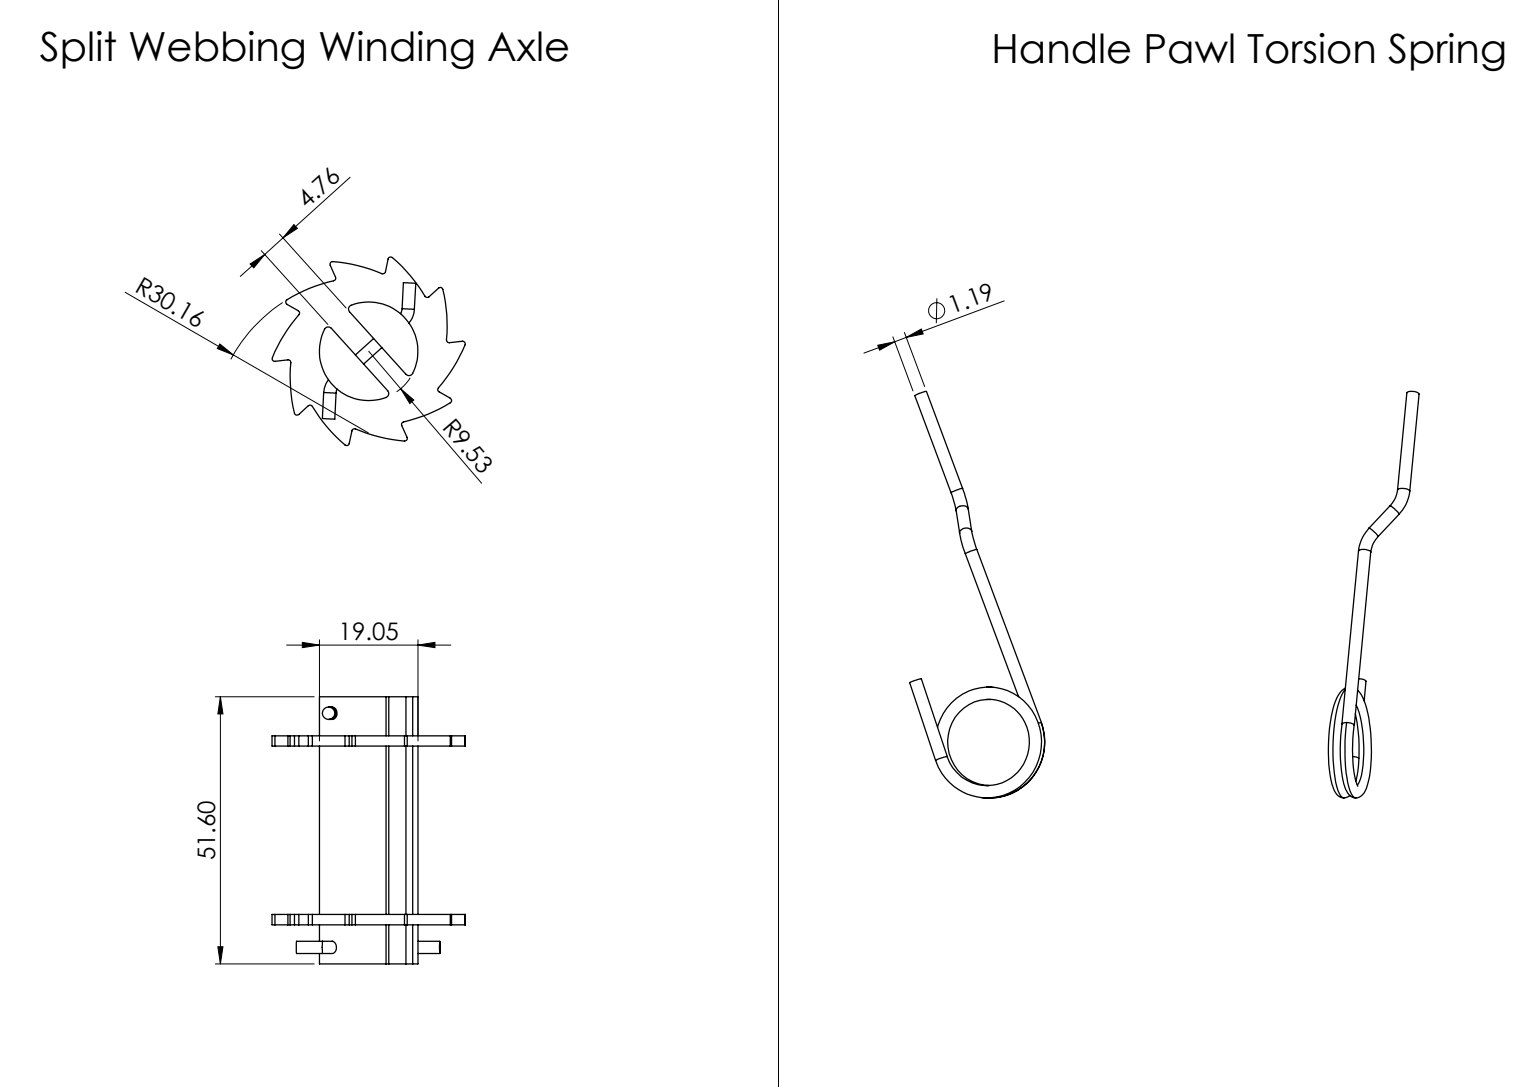
ISO-10303-21;
HEADER;
FILE_DESCRIPTION (('STEP AP214'),
    '1' );
FILE_NAME ('Handle Pawl Torsion Spring.step',
    '2026-10-09T14:10:49',
    ( '' ),
    ( '' ),
    'SwSTEP 2.0',
    'SolidWorks 2026',
    '' );
FILE_SCHEMA (( 'AUTOMOTIVE_DESIGN' ));
ENDSEC;

DATA;
#16=CARTESIAN_POINT ( 'NONE',  ( 20.19277141636333894, -1.028702071915735816, -14.77014087419847499 ) ) ;
#19=CARTESIAN_POINT ( 'NONE',  ( 10.74587282237300023, -3.551474423027108696, -17.13904648846254730 ) ) ;
#30=CARTESIAN_POINT ( 'NONE',  ( 16.87573345534896063, 1.342421174834532049, -14.70424319714138583 ) ) ;
#38=ADVANCED_FACE ( 'NONE', ( #13541 ), #20247, .T. ) ;
#40=CLOSED_SHELL ( 'NONE', ( #13341, #4807, #5036, #2626, #8435, #8593, #10298, #38, #14436, #19908, #617, #19403, #13246, #15792, #17350, #9101 ) ) ;
#47=CARTESIAN_POINT ( 'NONE',  ( 12.03790632155779505, -1.842118199788904453, -16.73074338374886594 ) ) ;
#86=CARTESIAN_POINT ( 'NONE',  ( 19.20082524333561125, -5.215953177437151034, -14.22689379871408022 ) ) ;
#131=CARTESIAN_POINT ( 'NONE',  ( 19.71883509336728224, 0.07040483093252521141, -14.88702419437599112 ) ) ;
#134=CARTESIAN_POINT ( 'NONE',  ( 18.64212857235120069, -7.698692359554816456, -15.50269025218566021 ) ) ;
#163=CARTESIAN_POINT ( 'NONE',  ( 13.41487274969213317, -6.317043706895210775, -16.60971403326354334 ) ) ;
#164=CARTESIAN_POINT ( 'NONE',  ( 14.93145837000203358, 15.36419388438619826, -20.01065317369261365 ) ) ;
#184=CARTESIAN_POINT ( 'NONE',  ( 14.93145837000203358, 15.36419388438619826, -20.01065317369261365 ) ) ;
#194=CARTESIAN_POINT ( 'NONE',  ( 13.97919557092905407, 2.287850299137407006, -16.10306415954642389 ) ) ;
#196=CARTESIAN_POINT ( 'NONE',  ( 19.79930818132203285, -2.883721276782408083, -14.18765533889165553 ) ) ;
#232=CARTESIAN_POINT ( 'NONE',  ( 9.410620405120566190, 30.63641399982339308, -22.17591973292933361 ) ) ;
#247=CARTESIAN_POINT ( 'NONE',  ( 11.07281055964317495, -1.101114635511414530, -16.96369225983369944 ) ) ;
#262=CARTESIAN_POINT ( 'NONE',  ( 18.00364882752649720, -8.167742914975729462, -14.89596189428242567 ) ) ;
#270=CARTESIAN_POINT ( 'NONE',  ( 14.14748371971443675, 0.7006734101483724775, -16.02524869538980212 ) ) ;
#288=VERTEX_POINT ( 'NONE', #14647 ) ;
#303=CARTESIAN_POINT ( 'NONE',  ( 12.81960190910725750, -6.042093227902952002, -15.51352245845575695 ) ) ;
#351=CARTESIAN_POINT ( 'NONE',  ( 20.07318776485353240, -0.6525838462317746780, -14.80377008654006055 ) ) ;
#356=CARTESIAN_POINT ( 'NONE',  ( 14.93741582401050394, -8.328813464873949357, -16.31187028222389657 ) ) ;
#384=CARTESIAN_POINT ( 'NONE',  ( 11.42192246508016140, -4.515843507428392023, -15.23392906717917228 ) ) ;
#394=FACE_OUTER_BOUND ( 'NONE', #19852, .T. ) ;
#416=CARTESIAN_POINT ( 'NONE',  ( 19.10984178700001479, -5.369063563745102741, -14.24189854854983217 ) ) ;
#432=EDGE_LOOP ( 'NONE', ( #13598, #21453 ) ) ;
#440=LINE ( 'NONE', #5512, #18865 ) ;
#472=CARTESIAN_POINT ( 'NONE',  ( 19.75964483560148466, 0.004337915005267487314, -14.87722094040863752 ) ) ;
#476=CARTESIAN_POINT ( 'NONE',  ( 17.01227936190448986, 2.147986159030752962, -15.15785924608550950 ) ) ;
#481=VECTOR ( 'NONE', #15576, 1000.000000000000000 ) ;
#484=CARTESIAN_POINT ( 'NONE',  ( 14.83746136476627520, -7.423169472682626058, -15.14267033774566684 ) ) ;
#515=CARTESIAN_POINT ( 'NONE',  ( 19.96989445820344855, -1.596441888161631573, -15.57706592207198781 ) ) ;
#529=CARTESIAN_POINT ( 'NONE',  ( 14.96245394991857580, -7.172648401804374352, -15.07977408558167731 ) ) ;
#537=CARTESIAN_POINT ( 'NONE',  ( 11.61240041076558960, -6.892588391211154963, -15.33507383697825688 ) ) ;
#573=EDGE_CURVE ( 'NONE', #9259, #10436, #9589, .T. ) ;
#583=CARTESIAN_POINT ( 'NONE',  ( 19.69663990328241354, 0.4662939914211877701, -14.34639758507740304 ) ) ;
#603=CARTESIAN_POINT ( 'NONE',  ( 14.47570345013334148, 0.8437009842499967327, -15.92338500342878937 ) ) ;
#604=CARTESIAN_POINT ( 'NONE',  ( 13.37471192292826139, 17.58265891940030556, -17.38954468002155451 ) ) ;
#617=ADVANCED_FACE ( 'NONE', ( #11371 ), #19429, .T. ) ;
#623=CARTESIAN_POINT ( 'NONE',  ( 19.10610158472843167, -0.2473655220616398365, -14.45733488498617625 ) ) ;
#624=VERTEX_POINT ( 'NONE', #4304 ) ;
#638=CARTESIAN_POINT ( 'NONE',  ( 11.79048631737284936, -6.033539481721004627, -16.29381363364702295 ) ) ;
#654=CARTESIAN_POINT ( 'NONE',  ( 11.56051848560380435, -4.566074003843849205, -16.36139799744035628 ) ) ;
#681=CARTESIAN_POINT ( 'NONE',  ( 14.14084833952063747, 15.36419388438619649, -16.93566361603518899 ) ) ;
#685=CARTESIAN_POINT ( 'NONE',  ( 12.15102624612472404, 0.6667575905376122991, -16.60929033701790303 ) ) ;
#703=DIRECTION ( 'NONE',  ( -0.4128958666089267981, 0.5884034904305870395, 0.6951966166390379787 ) ) ;
#707=CARTESIAN_POINT ( 'NONE',  ( 14.70048594802655550, 0.9231428247525146347, -15.85394111059815891 ) ) ;
#730=CARTESIAN_POINT ( 'NONE',  ( 11.61321856100838446, -3.658181173652626850, -15.64410391039172765 ) ) ;
#736=VERTEX_POINT ( 'NONE', #11907 ) ;
#767=CARTESIAN_POINT ( 'NONE',  ( 10.76290084369569300, -4.809670885807078911, -16.11272035331650088 ) ) ;
#769=CARTESIAN_POINT ( 'NONE',  ( 20.91979369334982053, -1.192140601152523738, -15.67394038340841433 ) ) ;
#778=AXIS2_PLACEMENT_3D ( 'NONE', #1408, #18118, #2976 ) ;
#797=EDGE_CURVE ( 'NONE', #13084, #13654, #10323, .T. ) ;
#802=CARTESIAN_POINT ( 'NONE',  ( 19.23564988699146383, 0.9575902230288153572, -14.49006204532864928 ) ) ;
#814=ORIENTED_EDGE ( 'NONE', *, *, #7876, .F. ) ;
#845=CARTESIAN_POINT ( 'NONE',  ( 12.49368766438004918, -5.659044190558311094, -16.93738714635493992 ) ) ;
#865=ORIENTED_EDGE ( 'NONE', *, *, #1285, .F. ) ;
#887=DIRECTION ( 'NONE',  ( -0.3482992169606098365, 0.9330960544336215357, -0.08955115110948595747 ) ) ;
#910=CARTESIAN_POINT ( 'NONE',  ( 12.58231226417771431, 1.068540657403270533, -16.47635048232419308 ) ) ;
#941=EDGE_LOOP ( 'NONE', ( #20654, #15170, #9199, #19380 ) ) ;
#947=CARTESIAN_POINT ( 'NONE',  ( 14.42288723307214937, 1.091498886294842929, -16.08015919209965361 ) ) ;
#963=ORIENTED_EDGE ( 'NONE', *, *, #13424, .F. ) ;
#1008=CARTESIAN_POINT ( 'NONE',  ( 20.27534158291089383, -5.683549201221528513, -13.95679996024211178 ) ) ;
#1036=DIRECTION ( 'NONE',  ( -0.3482992169606098365, 0.9330960544336215357, -0.08955115110948595747 ) ) ;
#1044=CARTESIAN_POINT ( 'NONE',  ( 19.83909275568333186, -0.5540471600307961264, -14.82645783518564109 ) ) ;
#1052=CARTESIAN_POINT ( 'NONE',  ( 19.96181834009323097, -0.9481503896113792074, -14.83657039408695510 ) ) ;
#1059=CARTESIAN_POINT ( 'NONE',  ( 20.09804786238122887, -3.027183637114436721, -15.33410839348449528 ) ) ;
#1069=CARTESIAN_POINT ( 'NONE',  ( 10.37745330590589177, -3.119969851305963271, -17.16587059559704187 ) ) ;
#1121=CARTESIAN_POINT ( 'NONE',  ( 20.12232975604240437, -5.942321916599345499, -13.98511480133279150 ) ) ;
#1160=CARTESIAN_POINT ( 'NONE',  ( 20.35972896993364856, -6.628739050289367718, -15.16768908211401801 ) ) ;
#1170=CARTESIAN_POINT ( 'NONE',  ( 11.16602196571547800, -3.114676983449079284, -17.69632302812056679 ) ) ;
#1177=CARTESIAN_POINT ( 'NONE',  ( 20.03340970562774004, -2.288172619315485878, -15.38567779163451910 ) ) ;
#1221=AXIS2_PLACEMENT_3D ( 'NONE', #2364, #9093, #3917 ) ;
#1231=CARTESIAN_POINT ( 'NONE',  ( 17.36619415103275088, -8.153771590782046275, -14.56055014027420036 ) ) ;
#1264=CARTESIAN_POINT ( 'NONE',  ( 19.90082682264116087, -1.596441870638235727, -15.30843464744698501 ) ) ;
#1272=CARTESIAN_POINT ( 'NONE',  ( 20.22951472560300346, -1.344520626714845069, -14.75553331646387711 ) ) ;
#1273=CARTESIAN_POINT ( 'NONE',  ( 11.59908291261232094, -3.110513798225231330, -17.38546622976265255 ) ) ;
#1285=EDGE_CURVE ( 'NONE', #736, #11912, #12594, .T. ) ;
#1291=CARTESIAN_POINT ( 'NONE',  ( 21.56164019270388721, -3.402113909207450604, -14.89232589754399072 ) ) ;
#1308=EDGE_CURVE ( 'NONE', #13225, #13084, #14235, .T. ) ;
#1333=CARTESIAN_POINT ( 'NONE',  ( 12.18257168130173085, -7.051347156841528907, -15.68602168311090317 ) ) ;
#1364=CARTESIAN_POINT ( 'NONE',  ( 12.49611771652354975, -6.111721726754139716, -15.44633277492886592 ) ) ;
#1366=CARTESIAN_POINT ( 'NONE',  ( 13.37471192292826139, 17.58265891940030556, -17.38954468002155451 ) ) ;
#1373=CARTESIAN_POINT ( 'NONE',  ( 20.12904150882413035, -1.237462911438615754, -14.78438767367360285 ) ) ;
#1381=ADVANCED_BREP_SHAPE_REPRESENTATION ( '', ( #20809, #2234 ), #4182 ) ;
#1404=EDGE_CURVE ( 'NONE', #5048, #5980, #5871, .T. ) ;
#1408=CARTESIAN_POINT ( 'NONE',  ( 12.76235139282079167, 21.25996874134203907, -20.69948241803004407 ) ) ;
#1414=ORIENTED_EDGE ( 'NONE', *, *, #9671, .F. ) ;
#1423=CIRCLE ( 'NONE', #8464, 0.5953125000000000222 ) ;
#1439=ORIENTED_EDGE ( 'NONE', *, *, #1863, .T. ) ;
#1442=CARTESIAN_POINT ( 'NONE',  ( 11.97174136233939556, 21.25996874134203551, -17.62449286037261942 ) ) ;
#1443=CARTESIAN_POINT ( 'NONE',  ( 15.38918027679277856, -8.419993694669582140, -14.99388312876912721 ) ) ;
#1479=CARTESIAN_POINT ( 'NONE',  ( 20.06462325295336413, -2.740908352756980193, -14.15992765561396105 ) ) ;
#1489=CARTESIAN_POINT ( 'NONE',  ( 20.36422011069876348, -6.543713029916194301, -15.61347904700674860 ) ) ;
#1491=STYLED_ITEM ( 'NONE', ( #1555 ), #20809 ) ;
#1497=CARTESIAN_POINT ( 'NONE',  ( 17.12726144548341267, -7.073893271879835964, -15.84366279292657609 ) ) ;
#1555=PRESENTATION_STYLE_ASSIGNMENT (( #13509 ) ) ;
#1580=CARTESIAN_POINT ( 'NONE',  ( 14.40215569916422922, -8.180188028388664989, -16.42876195537290585 ) ) ;
#1591=CARTESIAN_POINT ( 'NONE',  ( 10.89278871826026496, -3.741510472769750351, -15.20017649982984409 ) ) ;
#1595=CARTESIAN_POINT ( 'NONE',  ( 19.84534036711146143, -1.573540299197002224, -15.46898262837090243 ) ) ;
#1596=EDGE_LOOP ( 'NONE', ( #17698, #10706, #3633, #1414 ) ) ;
#1604=CARTESIAN_POINT ( 'NONE',  ( 14.65560158155272674, -7.011384195667019981, -16.35874738822244723 ) ) ;
#1654=FILL_AREA_STYLE ('',( #4874 ) ) ;
#1673=CARTESIAN_POINT ( 'NONE',  ( 20.18250336069275974, -0.9908562680277209767, -14.77328602232822519 ) ) ;
#1677=CARTESIAN_POINT ( 'NONE',  ( 10.97108191230651109, -4.649804219968682872, -17.12215967864936772 ) ) ;
#1687=CARTESIAN_POINT ( 'NONE',  ( 19.35144069079204954, -5.834156456616997666, -15.24901388582027195 ) ) ;
#1689=CARTESIAN_POINT ( 'NONE',  ( 20.53156612299923012, -1.359449706705494254, -15.90722162142133733 ) ) ;
#1697=CARTESIAN_POINT ( 'NONE',  ( 11.48491928014121122, -6.408048376592000217, -17.19675141021907550 ) ) ;
#1707=CARTESIAN_POINT ( 'NONE',  ( 12.66650400994676140, -5.505089894041057974, -16.74975958372730389 ) ) ;
#1708=FACE_OUTER_BOUND ( 'NONE', #17654, .T. ) ;
#1738=CARTESIAN_POINT ( 'NONE',  ( 9.321907506464571114, 3.084972983906390631, -16.32229253314513784 ) ) ;
#1741=CARTESIAN_POINT ( 'NONE',  ( 17.15398648756978517, -6.962794673133186230, -14.62314114746725302 ) ) ;
#1749=ORIENTED_EDGE ( 'NONE', *, *, #20617, .T. ) ;
#1783=CARTESIAN_POINT ( 'NONE',  ( 20.22951472560300346, -1.344520626714845069, -14.75553331646387711 ) ) ;
#1788=CARTESIAN_POINT ( 'NONE',  ( 14.12322331492428873, -8.081744716033297138, -16.48945220907392795 ) ) ;
#1793=AXIS2_PLACEMENT_3D ( 'NONE', #6813, #5365, #8679 ) ;
#1817=CARTESIAN_POINT ( 'NONE',  ( 14.52745126260834141, -6.964383640051551083, -16.38517187279768095 ) ) ;
#1818=CARTESIAN_POINT ( 'NONE',  ( 11.81489480681374715, -4.423560566030090513, -15.68132100509055782 ) ) ;
#1854=CARTESIAN_POINT ( 'NONE',  ( 12.37528884409636021, -5.524115550796262042, -15.59548877588442650 ) ) ;
#1863=EDGE_CURVE ( 'NONE', #11912, #13084, #7491, .T. ) ;
#1899=CARTESIAN_POINT ( 'NONE',  ( 10.88641682560997204, -1.671568469779255439, -17.03366785910728964 ) ) ;
#1910=LINE ( 'NONE', #1689, #10939 ) ;
#1912=ORIENTED_EDGE ( 'NONE', *, *, #1404, .T. ) ;
#1925=CARTESIAN_POINT ( 'NONE',  ( 12.99564195812022405, -0.1559143132144474864, -16.39129925056700543 ) ) ;
#1960=CARTESIAN_POINT ( 'NONE',  ( 13.22923918826351297, -6.405949669792143197, -15.43418026626714301 ) ) ;
#2006=CARTESIAN_POINT ( 'NONE',  ( 17.44897684999575915, -8.217241507614266638, -15.76094700865116138 ) ) ;
#2012=CARTESIAN_POINT ( 'NONE',  ( 12.46399079089267836, -5.664758814889668592, -16.85385019909982418 ) ) ;
#2028=CARTESIAN_POINT ( 'NONE',  ( 18.79169812173498144, -0.2733990383971263149, -14.58197954317160416 ) ) ;
#2029=CARTESIAN_POINT ( 'NONE',  ( 11.67873622359053165, -4.444366717925562149, -15.39547690709331995 ) ) ;
#2062=CARTESIAN_POINT ( 'NONE',  ( 19.41812612159816354, -4.815725606720878460, -14.19246007111251551 ) ) ;
#2067=DIRECTION ( 'NONE',  ( -0.9161599507719021540, -0.3242921320961419940, -0.2355537256384720723 ) ) ;
#2070=CARTESIAN_POINT ( 'NONE',  ( 14.59416852906185902, -8.664514012370643670, -15.20522331642918168 ) ) ;
#2116=CARTESIAN_POINT ( 'NONE',  ( 19.83642166017488151, -0.1294698813808727589, -14.85952381701978453 ) ) ;
#2121=CARTESIAN_POINT ( 'NONE',  ( 11.96169894293330138, 0.4392826198422947193, -16.66899426637521842 ) ) ;
#2142=CARTESIAN_POINT ( 'NONE',  ( 13.28268573882264469, 19.39178765922512326, -19.83174211820151100 ) ) ;
#2145=CARTESIAN_POINT ( 'NONE',  ( 16.67159889069950296, 1.010067806219507647, -15.24940416025467904 ) ) ;
#2181=CARTESIAN_POINT ( 'NONE',  ( 14.29938834594686448, -6.988883160487315394, -15.21728503260617593 ) ) ;
#2191=CARTESIAN_POINT ( 'NONE',  ( 21.25282423609957050, -2.645784314445630780, -13.67651348702517744 ) ) ;
#2199=AXIS2_PLACEMENT_3D ( 'NONE', #2142, #14330, #703 ) ;
#2234=AXIS2_PLACEMENT_3D ( 'NONE', #14022, #2275, #17644 ) ;
#2238=CARTESIAN_POINT ( 'NONE',  ( 14.08131258074581105, 1.962522422995664151, -16.02478678334940554 ) ) ;
#2253=CARTESIAN_POINT ( 'NONE',  ( 20.51985202635208694, -6.011610439988455568, -14.03095391611717346 ) ) ;
#2260=CARTESIAN_POINT ( 'NONE',  ( 19.84534036711146143, -1.573540299197002224, -15.46898262837090243 ) ) ;
#2261=CARTESIAN_POINT ( 'NONE',  ( 16.91309518241949661, 0.9412279162453636161, -15.17502221664437911 ) ) ;
#2275=DIRECTION ( 'NONE',  ( 0.000000000000000000, 0.000000000000000000, 1.000000000000000000 ) ) ;
#2280=CARTESIAN_POINT ( 'NONE',  ( 14.37256150657012199, 1.100706393900077407, -15.89788116173771648 ) ) ;
#2292=CARTESIAN_POINT ( 'NONE',  ( 20.36270583931112910, -6.627754957419618620, -15.18422494847827586 ) ) ;
#2300=CARTESIAN_POINT ( 'NONE',  ( 11.30427477552373894, 0.1855068411375157544, -16.71599931165275521 ) ) ;
#2319=TOROIDAL_SURFACE ( 'NONE', #21731, 3.174999999999999822, 0.5953125000000000222 ) ;
#2350=CARTESIAN_POINT ( 'NONE',  ( 12.80562560408363915, 1.259733001188390489, -16.40790845565960510 ) ) ;
#2364=CARTESIAN_POINT ( 'NONE',  ( 9.262381024405307528, 30.63641399982339308, -21.59935919086856515 ) ) ;
#2366=CARTESIAN_POINT ( 'NONE',  ( 11.33696792159741662, 0.1808088057320689224, -16.81606727879834651 ) ) ;
#2374=CARTESIAN_POINT ( 'NONE',  ( 12.56940319628321490, -0.6962962921986948217, -16.53391742796571151 ) ) ;
#2392=CARTESIAN_POINT ( 'NONE',  ( 19.33923522922928839, 0.3748380676697945502, -15.04264288269788885 ) ) ;
#2397=CARTESIAN_POINT ( 'NONE',  ( 14.55664670201521638, -7.269926523219644388, -16.33216676728327599 ) ) ;
#2431=CARTESIAN_POINT ( 'NONE',  ( 11.11706420665069217, -4.717387944073672124, -16.40916909168538496 ) ) ;
#2460=CARTESIAN_POINT ( 'NONE',  ( 20.82734621676318199, -1.850212124675815195, -13.95953525842948828 ) ) ;
#2475=CARTESIAN_POINT ( 'NONE',  ( 17.53455994494808223, -8.551185372775542248, -15.70422118946672363 ) ) ;
#2500=CARTESIAN_POINT ( 'NONE',  ( 19.39574039404867278, 0.4330848887872487118, -14.99545623812619866 ) ) ;
#2502=CARTESIAN_POINT ( 'NONE',  ( 19.50328736735570345, -0.8676315445611676447, -15.54195256409067483 ) ) ;
#2520=CARTESIAN_POINT ( 'NONE',  ( 10.63496985936944483, -4.911985970482035668, -15.93575590714733536 ) ) ;
#2531=AXIS2_PLACEMENT_3D ( 'NONE', #4319, #887, #5854 ) ;
#2571=CARTESIAN_POINT ( 'NONE',  ( 13.80933250118894229, 1.859310833520770867, -16.10574153504097694 ) ) ;
#2594=CARTESIAN_POINT ( 'NONE',  ( 19.84534036711146143, -1.573540299197002224, -15.46898262837090243 ) ) ;
#2616=CARTESIAN_POINT ( 'NONE',  ( 19.93134302918909384, -1.593178467216436411, -15.39176060413034364 ) ) ;
#2626=ADVANCED_FACE ( 'NONE', ( #13390 ), #3327, .T. ) ;
#2683=CARTESIAN_POINT ( 'NONE',  ( 20.38332674228396613, -1.359449706705494920, -15.33066107936057065 ) ) ;
#2684=CARTESIAN_POINT ( 'NONE',  ( 11.97511817037405812, -6.853367414429714977, -15.72877504999935283 ) ) ;
#2701=CARTESIAN_POINT ( 'NONE',  ( 19.84450919603384733, -1.527652306611041233, -14.98753281959816874 ) ) ;
#2711=CARTESIAN_POINT ( 'NONE',  ( 11.33771398496533855, 0.1030544890320075901, -16.36893042155433875 ) ) ;
#2715=( NAMED_UNIT ( * ) SI_UNIT ( $, .STERADIAN. ) SOLID_ANGLE_UNIT ( ) );
#2719=CARTESIAN_POINT ( 'NONE',  ( 19.49278356037279991, -0.05523789353248333145, -15.00694009703612686 ) ) ;
#2721=CARTESIAN_POINT ( 'NONE',  ( 17.19235063062528468, -7.334996653170583691, -15.79220656676793411 ) ) ;
#2730=CARTESIAN_POINT ( 'NONE',  ( 18.11264938600108820, 5.747448040522750823, -19.32386823132846132 ) ) ;
#2778=EDGE_LOOP ( 'NONE', ( #21084, #5570, #15508, #2989 ) ) ;
#2782=CARTESIAN_POINT ( 'NONE',  ( 11.87758290844151787, -6.747997337208533786, -15.74855984373561135 ) ) ;
#2812=CARTESIAN_POINT ( 'NONE',  ( 9.262381024405307528, 30.63641399982339308, -21.59935919086856515 ) ) ;
#2813=CARTESIAN_POINT ( 'NONE',  ( 20.07205047641097551, 0.5575362955879438198, -14.29572329288908605 ) ) ;
#2819=CARTESIAN_POINT ( 'NONE',  ( 17.77130180500099144, -8.167753660192959231, -13.99236777178278146 ) ) ;
#2827=CARTESIAN_POINT ( 'NONE',  ( 20.11644828361683324, -1.217489419619933066, -14.78816586879083772 ) ) ;
#2896=CARTESIAN_POINT ( 'NONE',  ( 20.18965527659050707, -5.828461386187921534, -13.97265621264273250 ) ) ;
#2930=CARTESIAN_POINT ( 'NONE',  ( 20.17509116920188106, -6.297343119843968218, -15.18573247873388610 ) ) ;
#2939=CARTESIAN_POINT ( 'NONE',  ( 14.41042916532441076, -7.397368266813621140, -15.94011715785100058 ) ) ;
#2947=CARTESIAN_POINT ( 'NONE',  ( 19.65610218525419484, -5.426016033732137700, -14.59150382834396886 ) ) ;
#2955=CARTESIAN_POINT ( 'NONE',  ( 19.16029575344082403, -5.702674460024825365, -15.43937346368577046 ) ) ;
#2963=CARTESIAN_POINT ( 'NONE',  ( 20.47011791841445216, -6.007381863893643370, -13.86582502354129254 ) ) ;
#2976=DIRECTION ( 'NONE',  ( -0.2490110332224855227, 0.000000000000000000, 0.9685006480810791629 ) ) ;
#2989=ORIENTED_EDGE ( 'NONE', *, *, #3460, .F. ) ;
#3009=CARTESIAN_POINT ( 'NONE',  ( 9.114141643690045314, 30.63641399982339308, -21.02279864880779670 ) ) ;
#3034=CARTESIAN_POINT ( 'NONE',  ( 21.19398735712951876, -3.814682859859762853, -15.02299825110072895 ) ) ;
#3043=CARTESIAN_POINT ( 'NONE',  ( 16.95410740259722004, 1.821792332331595432, -14.48457991158913494 ) ) ;
#3052=CARTESIAN_POINT ( 'NONE',  ( 19.52483535838462814, -0.1223081128681305918, -14.99489796488201421 ) ) ;
#3059=DIRECTION ( 'NONE',  ( -0.4128958666089267981, 0.5884034904305870395, 0.6951966166390379787 ) ) ;
#3102=CARTESIAN_POINT ( 'NONE',  ( 13.62051399351888747, 17.23237496650334677, -17.80340391586448234 ) ) ;
#3109=CARTESIAN_POINT ( 'NONE',  ( 12.88896270848683123, -7.596525905234238429, -15.53747963948190325 ) ) ;
#3144=CARTESIAN_POINT ( 'NONE',  ( 14.22429864969880065, 1.227399424245292137, -15.50635713965766982 ) ) ;
#3157=CARTESIAN_POINT ( 'NONE',  ( 16.37115362237207705, -7.227104028295391558, -16.00107671334114556 ) ) ;
#3162=CARTESIAN_POINT ( 'NONE',  ( 8.776506035771831193, 2.891917824018316097, -16.46252061043899673 ) ) ;
#3193=CARTESIAN_POINT ( 'NONE',  ( 19.78100715883822147, -2.554695793581883478, -14.20785545507690095 ) ) ;
#3247=CARTESIAN_POINT ( 'NONE',  ( 12.14585711117796230, -6.728073091731484823, -16.90832145949149279 ) ) ;
#3259=CARTESIAN_POINT ( 'NONE',  ( 17.12141331269406308, -7.465979233334057774, -15.36350049579159638 ) ) ;
#3271=CARTESIAN_POINT ( 'NONE',  ( 17.57968847865632611, -8.559078652989546399, -15.87053422043189421 ) ) ;
#3279=CARTESIAN_POINT ( 'NONE',  ( 17.54816828402311302, -6.930789574793553065, -15.75670520605582858 ) ) ;
#3310=CARTESIAN_POINT ( 'NONE',  ( 11.97174136233939556, 21.25996874134203551, -17.62449286037261942 ) ) ;
#3325=AXIS2_PLACEMENT_3D ( 'NONE', #21773, #6624, #15160 ) ;
#3327=CYLINDRICAL_SURFACE ( 'NONE', #3325, 0.5953125000000004663 ) ;
#3336=SURFACE_SIDE_STYLE ('',( #12058 ) ) ;
#3363=CARTESIAN_POINT ( 'NONE',  ( 11.30579500508379809, -5.488445583102078196, -17.06917961439425824 ) ) ;
#3368=CARTESIAN_POINT ( 'NONE',  ( 12.46105965416778716, -5.663837116554884865, -16.83730257442121214 ) ) ;
#3383=CARTESIAN_POINT ( 'NONE',  ( 11.89504694164775422, -2.569623862214921228, -16.80242428561735935 ) ) ;
#3413=CARTESIAN_POINT ( 'NONE',  ( 19.59062520529572993, -4.350225641996413373, -14.17140907119074988 ) ) ;
#3420=EDGE_CURVE ( 'NONE', #12389, #6378, #8643, .T. ) ;
#3435=( LENGTH_UNIT ( ) NAMED_UNIT ( * ) SI_UNIT ( .MILLI., .METRE. ) );
#3455=CARTESIAN_POINT ( 'NONE',  ( 20.21692672805859559, -1.125648057385024270, -14.76250352900288298 ) ) ;
#3458=CARTESIAN_POINT ( 'NONE',  ( 18.38276939006084731, -7.844924378857746738, -15.55834805662867737 ) ) ;
#3460=EDGE_CURVE ( 'NONE', #10436, #20642, #13949, .T. ) ;
#3469=CARTESIAN_POINT ( 'NONE',  ( 19.40594143866619703, -5.840264277364781265, -15.43021847716318717 ) ) ;
#3483=CARTESIAN_POINT ( 'NONE',  ( 11.99578385045931839, -4.049420365113250320, -16.84642447179846414 ) ) ;
#3485=CARTESIAN_POINT ( 'NONE',  ( 10.70549249095554423, -4.788864733378723315, -15.64570743106055062 ) ) ;
#3515=CARTESIAN_POINT ( 'NONE',  ( 10.40254502969509964, -3.119958055837774413, -17.26346415963410053 ) ) ;
#3517=CARTESIAN_POINT ( 'NONE',  ( 12.92878071497339931, -6.147102104778971565, -15.49261626134594572 ) ) ;
#3569=CARTESIAN_POINT ( 'NONE',  ( 10.77029199848827368, -2.261732460827042157, -17.08557667898591603 ) ) ;
#3571=CARTESIAN_POINT ( 'NONE',  ( 13.86631606410951534, 16.88209101360638797, -18.21726315170741017 ) ) ;
#3597=CARTESIAN_POINT ( 'NONE',  ( 17.98289846892998156, -6.707016923903890593, -15.66823201329469661 ) ) ;
#3631=CARTESIAN_POINT ( 'NONE',  ( 11.99812378058872930, -4.884789211543026255, -15.65751131229454352 ) ) ;
#3633=ORIENTED_EDGE ( 'NONE', *, *, #21383, .F. ) ;
#3678=CARTESIAN_POINT ( 'NONE',  ( 20.19361157104201965, -1.031857205123764887, -14.76988187127798113 ) ) ;
#3681=CARTESIAN_POINT ( 'NONE',  ( 14.52649824764486652, -8.218679500498163648, -16.40164373686755184 ) ) ;
#3689=CARTESIAN_POINT ( 'NONE',  ( 14.58173340751025471, -7.269924891899197661, -16.42976176385494469 ) ) ;
#3692=CIRCLE ( 'NONE', #1221, 0.5953125000000005773 ) ;
#3696=EDGE_CURVE ( 'NONE', #13654, #13907, #13968, .T. ) ;
#3707=CARTESIAN_POINT ( 'NONE',  ( 17.15392603081281564, 0.8698987389447586649, -15.10081136307826988 ) ) ;
#3743=CARTESIAN_POINT ( 'NONE',  ( 11.89701557769404339, -4.657576675299070601, -15.67185707629564106 ) ) ;
#3792=CARTESIAN_POINT ( 'NONE',  ( 15.20375925029796349, 2.251092030198116323, -15.69209066710536682 ) ) ;
#3815=CARTESIAN_POINT ( 'NONE',  ( 19.16641761350585327, -0.7858219696195261061, -14.45522876183969885 ) ) ;
#3850=CARTESIAN_POINT ( 'NONE',  ( 17.27833917726472635, -6.912512178730144008, -14.59757655905045937 ) ) ;
#3858=CARTESIAN_POINT ( 'NONE',  ( 17.28797397335993935, 2.432764323952259389, -15.11463947043034040 ) ) ;
#3904=CARTESIAN_POINT ( 'NONE',  ( 20.94764122044779597, -2.744589957913053269, -13.89552819659893146 ) ) ;
#3905=AXIS2_PLACEMENT_3D ( 'NONE', #164, #14011, #5237 ) ;
#3917=DIRECTION ( 'NONE',  ( -0.2490110332224855227, 0.000000000000000000, 0.9685006480810791629 ) ) ;
#3928=CARTESIAN_POINT ( 'NONE',  ( 20.23468942577036600, -1.359616646866762757, -14.75420580893919542 ) ) ;
#3940=EDGE_LOOP ( 'NONE', ( #17314, #10341, #7048, #8880, #865, #13918, #11787 ) ) ;
#3948=CARTESIAN_POINT ( 'NONE',  ( 20.08284348270143838, -2.741504599332891257, -14.26371703632316468 ) ) ;
#3967=CARTESIAN_POINT ( 'NONE',  ( 20.13189412415908564, -6.543715966850456311, -14.70988029850133927 ) ) ;
#3973=EDGE_CURVE ( 'NONE', #13907, #8439, #440, .T. ) ;
#4015=CARTESIAN_POINT ( 'NONE',  ( 14.63395006230149775, 2.144152496841746469, -15.86064623020511100 ) ) ;
#4036=CARTESIAN_POINT ( 'NONE',  ( 16.45009588711971560, 1.051937461999462364, -15.31736409357231388 ) ) ;
#4056=CARTESIAN_POINT ( 'NONE',  ( 19.35734219002929635, 0.4354800424330582675, -15.01894665276165242 ) ) ;
#4058=CARTESIAN_POINT ( 'NONE',  ( 19.41542498887948653, -5.356659253819461952, -14.11969569052875606 ) ) ;
#4071=ORIENTED_EDGE ( 'NONE', *, *, #19305, .F. ) ;
#4118=CARTESIAN_POINT ( 'NONE',  ( 12.35899892427300983, 0.8773483136192000709, -16.54479250898838671 ) ) ;
#4133=CARTESIAN_POINT ( 'NONE',  ( 20.10134609765169245, 0.5637867123784654488, -14.37936376174423359 ) ) ;
#4160=CARTESIAN_POINT ( 'NONE',  ( 19.34541047516490053, 0.4253635554462941171, -15.02868439565010839 ) ) ;
#4162=CARTESIAN_POINT ( 'NONE',  ( 11.73925543172950015, -4.504504147575669748, -15.65183323565414675 ) ) ;
#4182=( GEOMETRIC_REPRESENTATION_CONTEXT ( 3 ) GLOBAL_UNCERTAINTY_ASSIGNED_CONTEXT ( ( #5236 ) ) GLOBAL_UNIT_ASSIGNED_CONTEXT ( ( #6240, #11334, #2715 ) ) REPRESENTATION_CONTEXT ( 'NONE', 'WORKASPACE' ) );
#4228=CARTESIAN_POINT ( 'NONE',  ( 20.94643432978362441, -2.720492664379854819, -13.89672058998338855 ) ) ;
#4277=CARTESIAN_POINT ( 'NONE',  ( 20.04787453465361935, -2.740891176687007658, -14.09479187605280082 ) ) ;
#4291=CARTESIAN_POINT ( 'NONE',  ( 10.47583051940516619, -3.824893550810934517, -15.93653755199607147 ) ) ;
#4301=ORIENTED_EDGE ( 'NONE', *, *, #5314, .T. ) ;
#4304=CARTESIAN_POINT ( 'NONE',  ( 20.53156541068710439, -1.359447366214681985, -15.90722246059563361 ) ) ;
#4319=CARTESIAN_POINT ( 'NONE',  ( 12.76235139282079167, 21.25996874134203907, -20.69948241803004407 ) ) ;
#4342=CARTESIAN_POINT ( 'NONE',  ( 15.97930640409513536, -8.428197996455596197, -14.86420790539115444 ) ) ;
#4380=CARTESIAN_POINT ( 'NONE',  ( 21.32767659074639255, -3.394316947765121384, -14.52283687711769566 ) ) ;
#4387=CARTESIAN_POINT ( 'NONE',  ( 20.11003911965812208, -1.207134136194158103, -14.79009638531434589 ) ) ;
#4389=CARTESIAN_POINT ( 'NONE',  ( 12.34467035336512808, -0.5412634058883231125, -16.55697708178870897 ) ) ;
#4419=DIRECTION ( 'NONE',  ( -0.9037041334408598692, -0.3596272420165190220, -0.2323512126103423059 ) ) ;
#4454=CARTESIAN_POINT ( 'NONE',  ( 20.05076670763927282, -6.053556717652265995, -13.99866289979699197 ) ) ;
#4473=CARTESIAN_POINT ( 'NONE',  ( 20.53116362325268796, -1.359604737398370622, -15.90732750518314731 ) ) ;
#4482=CARTESIAN_POINT ( 'NONE',  ( 13.97450013175296490, 2.289333815574723374, -16.08697015436425559 ) ) ;
#4489=CARTESIAN_POINT ( 'NONE',  ( 19.38601130136307660, 0.1958779811795416381, -15.04182760293502241 ) ) ;
#4503=CARTESIAN_POINT ( 'NONE',  ( 20.47836239057684438, -0.2404636795067978394, -15.29125119441909497 ) ) ;
#4506=ORIENTED_EDGE ( 'NONE', *, *, #3973, .F. ) ;
#4511=EDGE_CURVE ( 'NONE', #6378, #624, #12988, .T. ) ;
#4513=B_SPLINE_CURVE_WITH_KNOTS ( 'NONE', 3,
 ( #16114, #10691, #7477, #17437, #15791, #2500, #14135, #5707, #12466, #19190, #4056, #4160, #10799, #17544, #2392, #10899, #9122, #14247, #17652, #20963, #9235, #4489, #9670, #16541, #18197, #21390, #2719, #17976, #3052, #16441, #9561, #4595, #14893, #8014, #8114, #16225, #18087, #16330, #7906, #1052, #11122, #4820, #11224, #12799, #18293, #4387, #2827, #1373, #11338, #17874, #6141, #9453, #13237, #1272 ),
 .UNSPECIFIED., .F., .F.,
 ( 4, 2, 2, 2, 2, 2, 2, 2, 2, 1, 2, 2, 2, 2, 2, 1, 1, 2, 2, 2, 2, 2, 2, 1, 2, 2, 2, 2, 4 ),
 ( 0.3951433275501288200, 0.4707511034793145921, 0.4896530474616097584, 0.4991040194527578411, 0.5038295054483319380, 0.5085549914439059238, 0.5180059634350532294, 0.5274569354262006460, 0.5463588794084951461, 0.5558098513996421186, 0.5605353373952158824, 0.5652608233907896462, 0.5841627673730825920, 0.6219666553376684837, 0.6408685993199608744, 0.6597705433022533761, 0.6975744312668370473, 0.7353783192314209405, 0.7542802632137127761, 0.7731822071960048337, 0.8487899831251725091, 0.8676919271074654549, 0.8771428990986118723, 0.8865938710897582897, 0.9243977590543427381, 0.9338487310454888224, 0.9432997030366349067, 0.9622016470189257431, 1.000005534983508193 ),
 .UNSPECIFIED. ) ;
#4578=CARTESIAN_POINT ( 'NONE',  ( 21.23025279753435512, -3.527030707732595083, -15.02425900349073018 ) ) ;
#4587=CARTESIAN_POINT ( 'NONE',  ( 20.36694164398600648, -3.336838402629868749, -14.76985127222394212 ) ) ;
#4593=EDGE_LOOP ( 'NONE', ( #8508, #9900 ) ) ;
#4595=CARTESIAN_POINT ( 'NONE',  ( 19.67322075098676137, -0.4140642647013181854, -14.93818290753014821 ) ) ;
#4603=CARTESIAN_POINT ( 'NONE',  ( 19.31280273682966353, -5.508750913041076558, -15.41181252894822862 ) ) ;
#4611=CARTESIAN_POINT ( 'NONE',  ( 20.33761533588227621, -6.627751949389748987, -15.08663078611084352 ) ) ;
#4633=FACE_OUTER_BOUND ( 'NONE', #6159, .T. ) ;
#4662=DIRECTION ( 'NONE',  ( 0.9037041334408600912, 0.3596272420165190775, 0.2323512126103423614 ) ) ;
#4663=CARTESIAN_POINT ( 'NONE',  ( 10.82333320179976432, -5.094404121093500493, -15.94728721271635585 ) ) ;
#4692=CARTESIAN_POINT ( 'NONE',  ( 20.89888763844149366, -4.983212492264129878, -15.05476727860177455 ) ) ;
#4703=DIRECTION ( 'NONE',  ( -0.2490110332224855227, 0.000000000000000000, 0.9685006480810791629 ) ) ;
#4705=CARTESIAN_POINT ( 'NONE',  ( 16.96554420789919604, 1.210820340708572029, -15.19753933136295032 ) ) ;
#4714=CARTESIAN_POINT ( 'NONE',  ( 20.11685381419291119, -5.681614476441408712, -14.67255263074746985 ) ) ;
#4726=DIRECTION ( 'NONE',  ( -0.3140771401027084853, 0.9459569826691583971, -0.08075231887918270235 ) ) ;
#4735=ORIENTED_EDGE ( 'NONE', *, *, #3420, .F. ) ;
#4739=ORIENTED_EDGE ( 'NONE', *, *, #20617, .F. ) ;
#4776=CARTESIAN_POINT ( 'NONE',  ( 19.40258015623733101, -6.852770372521438169, -14.12738853639282866 ) ) ;
#4802=CARTESIAN_POINT ( 'NONE',  ( 21.24987335672298627, -3.225771147898685243, -15.03024036818241527 ) ) ;
#4807=ADVANCED_FACE ( 'NONE', ( #15091 ), #2319, .T. ) ;
#4812=CARTESIAN_POINT ( 'NONE',  ( 14.53774918468628208, -7.260662509237028495, -16.24585327058502315 ) ) ;
#4820=CARTESIAN_POINT ( 'NONE',  ( 19.98755129532091601, -0.9945011873913147671, -14.82825913642804849 ) ) ;
#4827=CARTESIAN_POINT ( 'NONE',  ( 17.77073768271571197, -6.828400799270224475, -15.71113051208573808 ) ) ;
#4874=FILL_AREA_STYLE_COLOUR ( '', #17745 ) ;
#4903=CARTESIAN_POINT ( 'NONE',  ( 19.10022651896773027, -0.1605816450576252885, -14.01190017167833091 ) ) ;
#4915=CARTESIAN_POINT ( 'NONE',  ( 20.30414312236064234, -2.730712048100304656, -14.54529006522136569 ) ) ;
#4921=CARTESIAN_POINT ( 'NONE',  ( 13.23439868007747222, -6.150278290301139705, -16.64446557221927137 ) ) ;
#4961=ORIENTED_EDGE ( 'NONE', *, *, #4511, .F. ) ;
#5004=DIRECTION ( 'NONE',  ( 0.9037041334408598692, 0.3596272420165190220, 0.2323512126103423059 ) ) ;
#5005=CARTESIAN_POINT ( 'NONE',  ( 17.27816767801022024, -8.264717885962401311, -15.79824796366183648 ) ) ;
#5016=CARTESIAN_POINT ( 'NONE',  ( 19.78828714858439497, -5.681633152690531929, -13.39467244788724187 ) ) ;
#5024=CARTESIAN_POINT ( 'NONE',  ( 11.84474491476024482, -6.892609742072639989, -16.23866874929617055 ) ) ;
#5033=CARTESIAN_POINT ( 'NONE',  ( 12.69010466362585987, -5.538311079261389658, -16.74561394863653163 ) ) ;
#5036=ADVANCED_FACE ( 'NONE', ( #9079 ), #5661, .T. ) ;
#5048=VERTEX_POINT ( 'NONE', #6095 ) ;
#5069=CARTESIAN_POINT ( 'NONE',  ( 14.68361992452378573, -7.115731319896963392, -15.13783436087320666 ) ) ;
#5079=ORIENTED_EDGE ( 'NONE', *, *, #20823, .T. ) ;
#5113=CARTESIAN_POINT ( 'NONE',  ( 19.79101016780580125, -0.04868028894460403599, -14.86990150494959195 ) ) ;
#5115=CARTESIAN_POINT ( 'NONE',  ( 10.72409186464204112, -4.809670885807078022, -15.96177715662992824 ) ) ;
#5117=CARTESIAN_POINT ( 'NONE',  ( 19.58215480567678668, -6.970154277315572244, -15.30510421406360422 ) ) ;
#5124=CARTESIAN_POINT ( 'NONE',  ( 14.84133058652096082, -7.424716859588557760, -15.15897677154538670 ) ) ;
#5137=CARTESIAN_POINT ( 'NONE',  ( 18.77364033892985518, -6.130631416302358083, -15.51152502305813563 ) ) ;
#5138=CARTESIAN_POINT ( 'NONE',  ( 12.61411201210553124, 21.25996874134203907, -20.12292187596927562 ) ) ;
#5167=CARTESIAN_POINT ( 'NONE',  ( 19.79801356026766967, -2.842841826568478947, -14.18991051583819463 ) ) ;
#5204=DIRECTION ( 'NONE',  ( -0.3140771401027084853, 0.9459569826691583971, -0.08075231887918270235 ) ) ;
#5210=CARTESIAN_POINT ( 'NONE',  ( 20.02546805227182958, -0.5331770397073201107, -14.81556814719122528 ) ) ;
#5214=CARTESIAN_POINT ( 'NONE',  ( 10.77549486952163171, -3.766819462804153584, -17.13936903969156589 ) ) ;
#5222=CARTESIAN_POINT ( 'NONE',  ( 19.44050799006316055, -5.356675604303823945, -14.21729107038780704 ) ) ;
#5225=ORIENTED_EDGE ( 'NONE', *, *, #18561, .F. ) ;
#5227=DIRECTION ( 'NONE',  ( -0.1132953773954069598, 0.7241889112991808375, -0.6802312681817410667 ) ) ;
#5235=CARTESIAN_POINT ( 'NONE',  ( 16.61136152229415686, -7.189742716178133541, -15.95096700094411624 ) ) ;
#5236=UNCERTAINTY_MEASURE_WITH_UNIT (LENGTH_MEASURE( 1.000000000000000082E-05 ), #6240, 'distance_accuracy_value', 'NONE');
#5237=DIRECTION ( 'NONE',  ( 0.2490110332224869105, 8.271275069592406292E-16, -0.9685006480810787188 ) ) ;
#5267=CARTESIAN_POINT ( 'NONE',  ( 19.79304348009334547, -3.380154523412622236, -14.16596585955715781 ) ) ;
#5269=ORIENTED_EDGE ( 'NONE', *, *, #573, .T. ) ;
#5280=CIRCLE ( 'NONE', #21169, 0.5953125000000005773 ) ;
#5281=VECTOR ( 'NONE', #5569, 1000.000000000000000 ) ;
#5314=EDGE_CURVE ( 'NONE', #14268, #20548, #19814, .T. ) ;
#5322=CARTESIAN_POINT ( 'NONE',  ( 15.52272087797709332, -8.406786558832781253, -16.18343461258216465 ) ) ;
#5332=CARTESIAN_POINT ( 'NONE',  ( 11.63555623300968556, -3.657949307911554371, -15.72510360806348650 ) ) ;
#5343=CARTESIAN_POINT ( 'NONE',  ( 10.88152465653400469, -4.868500552888323618, -16.40605285604548413 ) ) ;
#5354=CARTESIAN_POINT ( 'NONE',  ( 19.00283808968254107, -0.5370937612277498774, -14.51149966347872677 ) ) ;
#5358=VECTOR ( 'NONE', #21416, 1000.000000000000000 ) ;
#5365=DIRECTION ( 'NONE',  ( -0.3482992169606098365, 0.9330960544336215357, -0.08955115110948595747 ) ) ;
#5386=CARTESIAN_POINT ( 'NONE',  ( 16.45317959916927109, -7.164694729300216558, -14.76837516743119849 ) ) ;
#5415=ORIENTED_EDGE ( 'NONE', *, *, #1285, .T. ) ;
#5431=CARTESIAN_POINT ( 'NONE',  ( 19.93069405542505379, -0.3168215820087039725, -14.83805648859174653 ) ) ;
#5435=CARTESIAN_POINT ( 'NONE',  ( 17.33536478547116033, -8.249904329601282171, -15.78574727907301067 ) ) ;
#5459=CARTESIAN_POINT ( 'NONE',  ( 16.90052181627606132, 0.9448800882039219973, -15.17889571493881107 ) ) ;
#5492=CARTESIAN_POINT ( 'NONE',  ( 19.80715417040793369, -3.131469232938576042, -14.17398794668478601 ) ) ;
#5500=CARTESIAN_POINT ( 'NONE',  ( 10.39684359234162692, -3.119971281104964689, -17.24762880647101682 ) ) ;
#5512=CARTESIAN_POINT ( 'NONE',  ( 13.86631606410951534, 16.88209101360638797, -18.21726315170741017 ) ) ;
#5540=CARTESIAN_POINT ( 'NONE',  ( 20.23338050908548880, -1.212044145622726443, -14.75678302155165511 ) ) ;
#5544=CARTESIAN_POINT ( 'NONE',  ( 16.36168651129493412, 2.265146188987181120, -15.35027226876440842 ) ) ;
#5553=CARTESIAN_POINT ( 'NONE',  ( 20.36530192851249410, -3.329039984996891910, -15.30396146910969968 ) ) ;
#5559=CARTESIAN_POINT ( 'NONE',  ( 10.51408890650479755, -3.826186581119058072, -16.12191821389345492 ) ) ;
#5569=DIRECTION ( 'NONE',  ( -0.3482992169606098365, 0.9330960544336215357, -0.08955115110948595747 ) ) ;
#5570=ORIENTED_EDGE ( 'NONE', *, *, #9400, .T. ) ;
#5587=CARTESIAN_POINT ( 'NONE',  ( 11.60094225694622772, -3.109384115592202402, -16.85129956413878816 ) ) ;
#5596=PRODUCT_DEFINITION ( 'UNKNOWN', '', #10181, #20483 ) ;
#5608=FACE_OUTER_BOUND ( 'NONE', #16059, .T. ) ;
#5611=CARTESIAN_POINT ( 'NONE',  ( 20.79919319928621846, -3.365577675197465535, -14.45920257639869355 ) ) ;
#5627=CARTESIAN_POINT ( 'NONE',  ( 19.75611402437074560, -4.719049260853012129, -15.34047214062004372 ) ) ;
#5661=CYLINDRICAL_SURFACE ( 'NONE', #8526, 0.5953124999999994671 ) ;
#5662=CARTESIAN_POINT ( 'NONE',  ( 17.19104467599775532, 2.097219702267779429, -15.10484033739021648 ) ) ;
#5686=CARTESIAN_POINT ( 'NONE',  ( 20.23508918937977796, -1.359453322992689506, -14.75410208910826704 ) ) ;
#5687=CARTESIAN_POINT ( 'NONE',  ( 13.72785506320953353, 0.4691747601981155480, -16.15643954551278938 ) ) ;
#5692=CARTESIAN_POINT ( 'NONE',  ( 21.29044094599970904, -2.646515516688929814, -13.86205913043574434 ) ) ;
#5707=CARTESIAN_POINT ( 'NONE',  ( 19.38236331922507816, 0.4371055082821885263, -15.00287587734002059 ) ) ;
#5710=CARTESIAN_POINT ( 'NONE',  ( 11.79490036187186597, -4.501343696292126495, -15.83274364649303578 ) ) ;
#5724=CARTESIAN_POINT ( 'NONE',  ( 11.35915110355360724, 0.1799203519520370387, -16.89710733764713879 ) ) ;
#5779=CARTESIAN_POINT ( 'NONE',  ( 13.29522536647246511, 1.581453584762025244, -16.25997556760552953 ) ) ;
#5803=CARTESIAN_POINT ( 'NONE',  ( 12.30151367325157530, -1.153126200941767543, -16.62801696922743844 ) ) ;
#5809=CARTESIAN_POINT ( 'NONE',  ( 17.95270069355080622, -8.291107314758558999, -14.47941694501537668 ) ) ;
#5810=ORIENTED_EDGE ( 'NONE', *, *, #5314, .F. ) ;
#5821=CARTESIAN_POINT ( 'NONE',  ( 17.43744253143330525, -7.133763992443639346, -14.52515173542417593 ) ) ;
#5846=DIRECTION ( 'NONE',  ( 0.9037041334408598692, 0.3596272420165190220, 0.2323512126103423059 ) ) ;
#5854=DIRECTION ( 'NONE',  ( -0.2490110332224855227, 0.000000000000000000, 0.9685006480810791629 ) ) ;
#5871=LINE ( 'NONE', #12863, #20210 ) ;
#5875=CARTESIAN_POINT ( 'NONE',  ( 16.83076340656427305, 2.188335711206311984, -15.21158537076933825 ) ) ;
#5896=CARTESIAN_POINT ( 'NONE',  ( 9.262381024405307528, 30.63641399982339308, -21.59935919086856515 ) ) ;
#5917=CARTESIAN_POINT ( 'NONE',  ( 19.50624135474398457, -0.8684152889774677808, -15.55849431363919599 ) ) ;
#5929=CARTESIAN_POINT ( 'NONE',  ( 20.46463427092750464, -6.006569699063351919, -13.84993367446087476 ) ) ;
#5979=CARTESIAN_POINT ( 'NONE',  ( 12.63934909048015598, -7.435355452895607620, -15.59063177402284239 ) ) ;
#5980=VERTEX_POINT ( 'NONE', #1738 ) ;
#6017=CARTESIAN_POINT ( 'NONE',  ( 14.09647384216111377, -8.336694694684233298, -16.02083815639807440 ) ) ;
#6028=EDGE_CURVE ( 'NONE', #288, #12389, #7133, .T. ) ;
#6030=CARTESIAN_POINT ( 'NONE',  ( 19.38382740634625279, -5.839277843515219502, -15.34916028355615225 ) ) ;
#6062=CIRCLE ( 'NONE', #19497, 3.770312499999998845 ) ;
#6095=CARTESIAN_POINT ( 'NONE',  ( 11.81489480681374715, -4.423560566030090513, -15.68132100509055782 ) ) ;
#6096=CARTESIAN_POINT ( 'NONE',  ( 16.27231063047230464, -8.394727124024923270, -14.79989961003369814 ) ) ;
#6132=CARTESIAN_POINT ( 'NONE',  ( 11.46521635664263172, -6.403241846889555333, -17.09334367148784750 ) ) ;
#6141=CARTESIAN_POINT ( 'NONE',  ( 20.17007366732797280, -1.298316440872414379, -14.77221745418293430 ) ) ;
#6150=CARTESIAN_POINT ( 'NONE',  ( 20.05951646036145064, -3.617492969892214916, -15.31622960476870077 ) ) ;
#6159=EDGE_LOOP ( 'NONE', ( #14102, #19969, #4301, #8895 ) ) ;
#6161=CARTESIAN_POINT ( 'NONE',  ( 11.62103910360368353, -6.985094744456809224, -15.76249710157855155 ) ) ;
#6203=CARTESIAN_POINT ( 'NONE',  ( 11.22892694877909037, -5.901286635516172829, -15.87608302377674363 ) ) ;
#6227=CARTESIAN_POINT ( 'NONE',  ( 20.35347976045076734, -6.056219266232003129, -15.15089302274523497 ) ) ;
#6240=( LENGTH_UNIT ( ) NAMED_UNIT ( * ) SI_UNIT ( .MILLI., .METRE. ) );
#6245=CARTESIAN_POINT ( 'NONE',  ( 14.87174356566636035, -8.043846378258365348, -15.78031415564158735 ) ) ;
#6251=CARTESIAN_POINT ( 'NONE',  ( 19.92745932268303477, -1.805445330691633155, -15.43621892734358525 ) ) ;
#6301=DIRECTION ( 'NONE',  ( -0.1132953773954069598, 0.7241889112991808375, -0.6802312681817410667 ) ) ;
#6308=CARTESIAN_POINT ( 'NONE',  ( 10.94429949547802217, -5.371352442010961958, -15.92721155031827429 ) ) ;
#6333=CARTESIAN_POINT ( 'NONE',  ( 20.08791609653252053, -6.411858537233912969, -15.20285343563792679 ) ) ;
#6343=CARTESIAN_POINT ( 'NONE',  ( 14.68672346071107171, -7.556859706525174580, -14.66503917285335845 ) ) ;
#6355=CARTESIAN_POINT ( 'NONE',  ( 21.12774895840593103, -3.365576380264218237, -15.73708478087671558 ) ) ;
#6370=CARTESIAN_POINT ( 'NONE',  ( 20.05229758337772594, 0.5585561380493306860, -14.21405859630069912 ) ) ;
#6378=VERTEX_POINT ( 'NONE', #1595 ) ;
#6422=CARTESIAN_POINT ( 'NONE',  ( 16.56531485685111349, -8.361256251594079814, -14.73559131467589545 ) ) ;
#6449=CIRCLE ( 'NONE', #2199, 0.5953125000000004663 ) ;
#6453=CARTESIAN_POINT ( 'NONE',  ( 21.24976161462477364, -2.911874215672294319, -15.04173616848670036 ) ) ;
#6456=PLANE ( 'NONE',  #11376 ) ;
#6465=CARTESIAN_POINT ( 'NONE',  ( 20.30874841272881781, -3.328473208352423995, -15.12328466456706266 ) ) ;
#6475=CARTESIAN_POINT ( 'NONE',  ( 21.04230988742212460, -1.217322810690986357, -15.63980871831360098 ) ) ;
#6481=CARTESIAN_POINT ( 'NONE',  ( 12.73876125567402084, -5.603651328527227804, -16.73694851094560221 ) ) ;
#6482=CARTESIAN_POINT ( 'NONE',  ( 13.62051399351888747, 17.23237496650334677, -17.80340391586448234 ) ) ;
#6570=CARTESIAN_POINT ( 'NONE',  ( 17.38294349214931245, -7.258570677684963002, -14.09221851007123227 ) ) ;
#6578=CARTESIAN_POINT ( 'NONE',  ( 12.46160258925475794, -5.743475608960900480, -17.28410787521212555 ) ) ;
#6586=CARTESIAN_POINT ( 'NONE',  ( 12.44019961867567936, -5.159552288755423710, -16.78848910152690621 ) ) ;
#6602=ORIENTED_EDGE ( 'NONE', *, *, #16336, .F. ) ;
#6624=DIRECTION ( 'NONE',  ( -0.1132953773954069598, 0.7241889112991808375, -0.6802312681817410667 ) ) ;
#6648=EDGE_CURVE ( 'NONE', #5980, #19395, #1423, .T. ) ;
#6659=CARTESIAN_POINT ( 'NONE',  ( 11.75816929971251135, -6.239310308105337377, -16.98506567453073401 ) ) ;
#6669=CARTESIAN_POINT ( 'NONE',  ( 19.47373669678540509, -0.8724954979520347376, -15.45837838233364003 ) ) ;
#6680=CARTESIAN_POINT ( 'NONE',  ( 10.63672918265855394, -3.118840168672979640, -17.63289682993426766 ) ) ;
#6689=CARTESIAN_POINT ( 'NONE',  ( 15.64213961604280279, -7.230076693056714632, -16.15356297515639383 ) ) ;
#6690=CYLINDRICAL_SURFACE ( 'NONE', #11661, 0.5953125000000004663 ) ;
#6766=CARTESIAN_POINT ( 'NONE',  ( 19.76004621270132589, 0.003678105342030234953, -14.87712536579863887 ) ) ;
#6769=CARTESIAN_POINT ( 'NONE',  ( 11.05988272033677333, -4.938043300071689679, -17.11035408892384524 ) ) ;
#6782=CARTESIAN_POINT ( 'NONE',  ( 14.35383053111052476, 1.091503432583336153, -15.81152456092466174 ) ) ;
#6801=CARTESIAN_POINT ( 'NONE',  ( 12.11282701178822307, -1.606571398329030620, -16.69983038620819826 ) ) ;
#6813=CARTESIAN_POINT ( 'NONE',  ( 20.38332674228396613, -1.359449706705494920, -15.33066107936057065 ) ) ;
#6835=CARTESIAN_POINT ( 'NONE',  ( 13.03688366823242539, 19.74207161212150297, -19.41788288235926885 ) ) ;
#6837=CARTESIAN_POINT ( 'NONE',  ( 19.23620902706707625, -5.156408013795760858, -14.22105839913137437 ) ) ;
#6873=DIRECTION ( 'NONE',  ( -0.9037041334408600912, -0.3596272420165190775, -0.2323512126103423614 ) ) ;
#6883=CARTESIAN_POINT ( 'NONE',  ( 20.01429352998429323, -0.5059105927738452024, -14.81829418944272980 ) ) ;
#6886=CARTESIAN_POINT ( 'NONE',  ( 16.40614462543630836, -8.411149092273442207, -15.98937562035452409 ) ) ;
#6891=CARTESIAN_POINT ( 'NONE',  ( 11.62603409302100133, -3.109374932586516316, -16.94889309930612598 ) ) ;
#6908=CARTESIAN_POINT ( 'NONE',  ( 11.88130483305368656, -3.258360441252182493, -16.83834492875844546 ) ) ;
#6936=CARTESIAN_POINT ( 'NONE',  ( 17.29174454768425306, 2.431241120636982167, -15.13097126745110721 ) ) ;
#6938=CARTESIAN_POINT ( 'NONE',  ( 19.51444747994706930, -4.586276125266755876, -14.17934498840143931 ) ) ;
#6985=CARTESIAN_POINT ( 'NONE',  ( 11.17732588453249676, -0.8204807644301946867, -16.92579435541830080 ) ) ;
#7012=CARTESIAN_POINT ( 'NONE',  ( 11.26403972753813498, -4.566074002652793062, -15.20827691245368563 ) ) ;
#7046=CARTESIAN_POINT ( 'NONE',  ( 19.00900242689141351, -5.516070221694524989, -14.25943734768673643 ) ) ;
#7048=ORIENTED_EDGE ( 'NONE', *, *, #18053, .F. ) ;
#7058=EDGE_LOOP ( 'NONE', ( #13050, #5269, #6602, #10827 ) ) ;
#7104=CARTESIAN_POINT ( 'NONE',  ( 13.29287104629461780, -7.674283192410473298, -16.66854283075998566 ) ) ;
#7125=CARTESIAN_POINT ( 'NONE',  ( 14.72818571777967911, -8.530828868335872173, -15.61771171534634917 ) ) ;
#7133=B_SPLINE_CURVE_WITH_KNOTS ( 'NONE', 3,
 ( #20970, #9459, #12580, #7698, #11127 ),
 .UNSPECIFIED., .F., .F.,
 ( 4, 1, 4 ),
 ( 0.000000000000000000, 0.2499992869893835068, 0.4992858149431267933 ),
 .UNSPECIFIED. ) ;
#7135=CARTESIAN_POINT ( 'NONE',  ( 12.56202611117371681, -0.7075020235198306029, -16.53645491934344136 ) ) ;
#7170=CARTESIAN_POINT ( 'NONE',  ( 18.39572628222328277, -6.194563955895442398, -14.37377832747673168 ) ) ;
#7178=CARTESIAN_POINT ( 'NONE',  ( 11.41584562260435476, -6.408040714559842144, -16.92812135191189071 ) ) ;
#7230=CARTESIAN_POINT ( 'NONE',  ( 19.00809320208830044, 1.143335664616400571, -14.55959509790053730 ) ) ;
#7237=CARTESIAN_POINT ( 'NONE',  ( 12.53629344102889043, -6.118443352698756499, -15.63122047053925812 ) ) ;
#7267=CARTESIAN_POINT ( 'NONE',  ( 12.44431693874740041, -5.663843069250676265, -16.77216482461518865 ) ) ;
#7276=CARTESIAN_POINT ( 'NONE',  ( 20.50345441762315346, -0.2404631712157635770, -15.38884510733137567 ) ) ;
#7278=CARTESIAN_POINT ( 'NONE',  ( 19.66680293064437279, -4.114175158726030013, -14.16347315398008888 ) ) ;
#7285=CARTESIAN_POINT ( 'NONE',  ( 11.35372246689305875, 0.1808204478124068870, -16.88120184474271213 ) ) ;
#7327=CARTESIAN_POINT ( 'NONE',  ( 20.31958935979195857, -0.4446614350344761935, -14.14521446648425851 ) ) ;
#7332=DIRECTION ( 'NONE',  ( -0.3140771401027084853, 0.9459569826691583971, -0.08075231887918270235 ) ) ;
#7348=CARTESIAN_POINT ( 'NONE',  ( 17.80163320068923838, 0.5619476608638845905, -14.89932917514400224 ) ) ;
#7360=ORIENTED_EDGE ( 'NONE', *, *, #10159, .F. ) ;
#7363=AXIS2_PLACEMENT_3D ( 'NONE', #15207, #5227, #10324 ) ;
#7367=CARTESIAN_POINT ( 'NONE',  ( 20.04522676934494640, -2.740773359176641666, -14.07817139380126292 ) ) ;
#7373=EDGE_LOOP ( 'NONE', ( #15734, #14065, #21143, #5810 ) ) ;
#7377=CARTESIAN_POINT ( 'NONE',  ( 14.18258613239171062, -8.464138069599565384, -16.53238645035581911 ) ) ;
#7388=CARTESIAN_POINT ( 'NONE',  ( 10.60440690384716156, -4.915117656754341979, -15.85244087925699930 ) ) ;
#7400=CARTESIAN_POINT ( 'NONE',  ( 11.27494694361443628, -4.667157449014243120, -16.43482124609427686 ) ) ;
#7430=CARTESIAN_POINT ( 'NONE',  ( 15.78242036309661067, 2.283158471184189242, -15.52125926898847652 ) ) ;
#7456=CARTESIAN_POINT ( 'NONE',  ( 13.16124604336415338, 0.02081130280650461684, -16.33707070753825263 ) ) ;
#7470=CARTESIAN_POINT ( 'NONE',  ( 12.76235139282079167, 21.25996874134203907, -20.69948241803004407 ) ) ;
#7477=CARTESIAN_POINT ( 'NONE',  ( 19.50032822304632063, 0.3607342948534012494, -14.94848289734256852 ) ) ;
#7480=CARTESIAN_POINT ( 'NONE',  ( 16.98959876662204849, 1.202893068749029126, -15.29982850647945369 ) ) ;
#7491=LINE ( 'NONE', #20849, #481 ) ;
#7518=CARTESIAN_POINT ( 'NONE',  ( 10.72409186464205355, -4.809670885807086016, -15.96177715662992824 ) ) ;
#7549=CARTESIAN_POINT ( 'NONE',  ( 11.50671703646502131, -0.1979220242447447820, -16.81508318434922344 ) ) ;
#7563=CARTESIAN_POINT ( 'NONE',  ( 11.44847493648600611, -6.403249497899589748, -17.02820558865678535 ) ) ;
#7572=DIRECTION ( 'NONE',  ( -0.4128958666089267981, 0.5884034904305870395, 0.6951966166390379787 ) ) ;
#7591=CARTESIAN_POINT ( 'NONE',  ( 11.61881240165799944, -3.657972840441829465, -15.65996692772725041 ) ) ;
#7651=CARTESIAN_POINT ( 'NONE',  ( 13.54613991325937583, 1.731347537946924309, -16.18443696118438524 ) ) ;
#7679=CARTESIAN_POINT ( 'NONE',  ( 20.48971467568342675, -6.006590701077150207, -13.94752972188701534 ) ) ;
#7694=CARTESIAN_POINT ( 'NONE',  ( 17.47713756659358353, -7.126243325886450819, -14.69286177225622225 ) ) ;
#7698=CARTESIAN_POINT ( 'NONE',  ( 20.37526559019908134, -1.303711368126346581, -14.71844211684304504 ) ) ;
#7708=CARTESIAN_POINT ( 'NONE',  ( 21.26534678900696562, -2.646493446368754388, -13.76446654770388811 ) ) ;
#7718=CIRCLE ( 'NONE', #7363, 0.5953125000000004663 ) ;
#7736=CYLINDRICAL_SURFACE ( 'NONE', #2531, 0.5953125000000005773 ) ;
#7757=CARTESIAN_POINT ( 'NONE',  ( 18.96717912055868638, -7.261914202138213703, -14.21728248528548200 ) ) ;
#7781=CARTESIAN_POINT ( 'NONE',  ( 20.99038978835910640, -4.695846652395300858, -15.04226715606432663 ) ) ;
#7785=DIRECTION ( 'NONE',  ( -0.2490110332224869660, -9.093548366658288884E-16, 0.9685006480810788299 ) ) ;
#7789=CARTESIAN_POINT ( 'NONE',  ( 20.32941413478750547, -1.382799517810166856, -14.66025672376848910 ) ) ;
#7805=CARTESIAN_POINT ( 'NONE',  ( 20.09493269590303655, -3.218164174955788326, -15.32593859137127090 ) ) ;
#7864=CARTESIAN_POINT ( 'NONE',  ( 14.56022883136782298, -8.303717150559636551, -15.17570085620177878 ) ) ;
#7876=EDGE_CURVE ( 'NONE', #19395, #5980, #13127, .T. ) ;
#7889=CARTESIAN_POINT ( 'NONE',  ( 20.07682953892606648, -1.527641563098319333, -15.89113342295757292 ) ) ;
#7896=ORIENTED_EDGE ( 'NONE', *, *, #10159, .T. ) ;
#7899=CARTESIAN_POINT ( 'NONE',  ( 14.17791483913661388, -8.465630425894779876, -16.51628623702010401 ) ) ;
#7906=CARTESIAN_POINT ( 'NONE',  ( 19.94878033733339606, -0.9245715916927551570, -14.84082521870049476 ) ) ;
#7909=B_SPLINE_SURFACE_WITH_KNOTS ( 'NONE', 3, 3, ( 
 ( #2502, #2616, #10692, #12577, #10800, #2397, #17440, #5587, #21066, #2280, #9236, #19300, #7367, #4058, #9347, #9018, #19194, #4162, #730 ),
 ( #5917, #11123, #21172, #6030, #2721, #15794, #7267, #10904, #4389, #17875, #16016, #623, #4277, #17546, #5821, #17653, #14137, #15688, #7591 ),
 ( #19524, #515, #14027, #11014, #20839, #20732, #845, #15905, #12348, #947, #7480, #19073, #3948, #14351, #7694, #14249, #16117, #5710, #12680 ),
 ( #19404, #12468, #9125, #14455, #20966, #17770, #6578, #1273, #19948, #20044, #16332, #11340, #4915, #2947, #16543, #18396, #18201, #13342, #21726 ),
 ( #16226, #8016, #6355, #14573, #14685, #19839, #11227, #1170, #7910, #18295, #21392, #9675, #16443, #4714, #8117, #6245, #21497, #9878, #13239 ),
 ( #14897, #6475, #16644, #1489, #8236, #15009, #15329, #6680, #18610, #20474, #13661, #10327, #8661, #17180, #262, #7125, #5024, #5343, #20593 ),
 ( #18508, #15109, #12215, #10107, #3271, #21828, #1697, #13442, #16093, #20704, #14107, #4133, #17517, #2253, #9204, #17288, #15661, #14002, #5559 ),
 ( #12317, #10874, #10664, #15770, #2475, #20810, #7563, #12440, #2366, #16239, #12693, #6370, #11240, #2963, #9689, #19313, #16455, #14702, #14363 ),
 ( #4503, #19540, #1291, #4611, #11139, #14805, #10918, #1069, #11356, #17887, #19737, #19417, #7708, #5929, #21079, #21405, #6161, #2520, #4291 ) ),
 .UNSPECIFIED., .F., .F., .F.,
 ( 4, 1, 1, 1, 1, 1, 4 ),
 ( 4, 1, 1, 1, 1, 1, 1, 1, 1, 1, 1, 1, 1, 1, 1, 1, 4 ),
 ( -0.01351613576970000022, 0.000000000000000000, 0.1250000000000000000, 0.2500000000000000000, 0.3750000000000000000, 0.5000000000000000000, 0.5135161357697000106 ),
 ( -0.02000000026063999958, 0.04500000058643999906, 0.1100000014334999998, 0.1750000022806000033, 0.2400000031276999790, 0.3050000039747000069, 0.3700000048218000104, 0.4350000056689000139, 0.5000000065160000728, 0.5650000073629999342, 0.6300000082101000487, 0.6950000090572000522, 0.7600000099042999446, 0.8250000107513000280, 0.8900000115984000315, 0.9550000124454999240, 1.020000013293000052 ),
 .UNSPECIFIED. ) ;
#7910=CARTESIAN_POINT ( 'NONE',  ( 12.01347082551317769, -0.1802273000781166867, -17.35803166960114652 ) ) ;
#7918=CARTESIAN_POINT ( 'NONE',  ( 19.52926446840631769, -5.159662720637996358, -15.37549714948907287 ) ) ;
#7974=CARTESIAN_POINT ( 'NONE',  ( 15.68359214062586560, -8.436795285945176914, -14.92921296275496701 ) ) ;
#8007=CARTESIAN_POINT ( 'NONE',  ( 20.50355652906860371, -2.693653029022725853, -13.33117366251859082 ) ) ;
#8014=CARTESIAN_POINT ( 'NONE',  ( 19.72907204108386381, -0.5191967632752201300, -14.91740567612944623 ) ) ;
#8016=CARTESIAN_POINT ( 'NONE',  ( 20.65797006290371840, -1.382799537871407747, -15.93813883736856418 ) ) ;
#8106=CARTESIAN_POINT ( 'NONE',  ( 12.76235139282079167, 21.25996874134203907, -20.69948241803004407 ) ) ;
#8107=CARTESIAN_POINT ( 'NONE',  ( 19.52298845727983689, -0.8684148934049937818, -15.62363129117676941 ) ) ;
#8114=CARTESIAN_POINT ( 'NONE',  ( 19.75485755962498757, -0.5674586355576572982, -14.90795299099519511 ) ) ;
#8117=CARTESIAN_POINT ( 'NONE',  ( 17.85758357290024634, -7.713152382332621571, -15.13302928010427273 ) ) ;
#8125=CARTESIAN_POINT ( 'NONE',  ( 18.19505925514423339, -6.585633048537570033, -15.62533351450368002 ) ) ;
#8126=FACE_OUTER_BOUND ( 'NONE', #10582, .T. ) ;
#8190=CARTESIAN_POINT ( 'NONE',  ( 18.48619651389723728, -7.612366584258952962, -14.31889584327733367 ) ) ;
#8208=AXIS2_PLACEMENT_3D ( 'NONE', #184, #21857, #11586 ) ;
#8226=CARTESIAN_POINT ( 'NONE',  ( 17.45417163489883805, -7.133772557271947257, -14.59029241586745940 ) ) ;
#8236=CARTESIAN_POINT ( 'NONE',  ( 17.62224048108546626, -8.420204368612866475, -16.19806502325979025 ) ) ;
#8242=CARTESIAN_POINT ( 'NONE',  ( 14.02148737346195162, -6.731876932532799174, -16.48869785773486640 ) ) ;
#8274=CARTESIAN_POINT ( 'NONE',  ( 19.79362740382113728, -2.761185752867874932, -14.19488287356966971 ) ) ;
#8321=CARTESIAN_POINT ( 'NONE',  ( 13.55088323884965718, -7.823075611188723855, -16.61323137860442856 ) ) ;
#8333=CARTESIAN_POINT ( 'NONE',  ( 11.38821987747605391, -3.675948036407177710, -15.27230885423398199 ) ) ;
#8345=CARTESIAN_POINT ( 'NONE',  ( 16.95801165930927823, -7.124051013253036579, -15.87873232967992543 ) ) ;
#8413=CARTESIAN_POINT ( 'NONE',  ( 20.10279225084434174, -0.7360295338183041602, -14.79594426830372278 ) ) ;
#8417=CARTESIAN_POINT ( 'NONE',  ( 10.88228110427572659, -4.361565139864056029, -17.13396526837493994 ) ) ;
#8426=CARTESIAN_POINT ( 'NONE',  ( 19.07381010491119255, -0.2526079255638566390, -14.35716343207643675 ) ) ;
#8435=ADVANCED_FACE ( 'NONE', ( #21007 ), #7736, .T. ) ;
#8439=VERTEX_POINT ( 'NONE', #21105 ) ;
#8446=CARTESIAN_POINT ( 'NONE',  ( 17.31838635957196715, -7.011879312349825533, -15.80413428893090355 ) ) ;
#8447=CARTESIAN_POINT ( 'NONE',  ( 10.68528288545773641, -4.809670885807078022, -15.81083395943519854 ) ) ;
#8464=AXIS2_PLACEMENT_3D ( 'NONE', #20014, #5204, #13524 ) ;
#8480=CARTESIAN_POINT ( 'NONE',  ( 15.24277482227980407, -7.221304072066160096, -15.02133152971018326 ) ) ;
#8508=ORIENTED_EDGE ( 'NONE', *, *, #16336, .T. ) ;
#8518=CARTESIAN_POINT ( 'NONE',  ( 14.93145837000203358, 15.36419388438619826, -20.01065317369261365 ) ) ;
#8526=AXIS2_PLACEMENT_3D ( 'NONE', #2683, #15755, #14311 ) ;
#8528=CARTESIAN_POINT ( 'NONE',  ( 20.19045750888530577, -1.020013971529757368, -14.77085460577932885 ) ) ;
#8531=CARTESIAN_POINT ( 'NONE',  ( 11.42902352243642028, -5.736415193692209868, -17.04764026735380611 ) ) ;
#8559=CARTESIAN_POINT ( 'NONE',  ( 11.89249479014546473, -3.409559102863189750, -16.84257439245622834 ) ) ;
#8593=ADVANCED_FACE ( 'NONE', ( #5608 ), #20303, .T. ) ;
#8595=CARTESIAN_POINT ( 'NONE',  ( 19.27010264103424930, -5.095940111084548363, -14.21560613677654317 ) ) ;
#8643=B_SPLINE_CURVE_WITH_KNOTS ( 'NONE', 3,
 ( #5686, #3928, #12447, #2701, #9000, #2260 ),
 .UNSPECIFIED., .F., .F.,
 ( 4, 1, 1, 4 ),
 ( 0.4992858149431267933, 0.5000000202745523703, 0.7500007535597175146, 1.000000000000000000 ),
 .UNSPECIFIED. ) ;
#8644=CARTESIAN_POINT ( 'NONE',  ( 19.67909734877197891, 0.1298811790940870847, -14.89708569419555317 ) ) ;
#8647=CARTESIAN_POINT ( 'NONE',  ( 17.89770978039528515, -8.066346848044377182, -15.66321486863013490 ) ) ;
#8653=CARTESIAN_POINT ( 'NONE',  ( 19.12821060939544182, -0.2463727629768049099, -14.53839379697989465 ) ) ;
#8661=CARTESIAN_POINT ( 'NONE',  ( 21.26384696840964494, -2.656554757447519677, -14.29854077623973296 ) ) ;
#8669=CARTESIAN_POINT ( 'NONE',  ( 15.51594691092190281, 1.079619396839424539, -15.60350270339164602 ) ) ;
#8670=CARTESIAN_POINT ( 'NONE',  ( 10.72409186464205355, -4.809670885807086016, -15.96177715662992824 ) ) ;
#8679=DIRECTION ( 'NONE',  ( -0.2490110332224889089, -7.284927983104707832E-16, 0.9685006480810781637 ) ) ;
#8698=CARTESIAN_POINT ( 'NONE',  ( 15.00318546702699152, -7.179718225927687492, -15.07128219575455219 ) ) ;
#8742=CARTESIAN_POINT ( 'NONE',  ( 19.96125241592742938, -0.3821940830726566762, -14.83098244249484310 ) ) ;
#8746=CARTESIAN_POINT ( 'NONE',  ( 17.39231329963745409, -8.234078972146175346, -15.77331051030036235 ) ) ;
#8770=CARTESIAN_POINT ( 'NONE',  ( 12.55470403860302753, -0.7187473132079236215, -16.53897826650729286 ) ) ;
#8803=CARTESIAN_POINT ( 'NONE',  ( 11.81489480681374715, -4.423560566030090513, -15.68132100509055782 ) ) ;
#8811=CARTESIAN_POINT ( 'NONE',  ( 11.44793084563043095, -6.323609490084446172, -16.58140058502533520 ) ) ;
#8834=CARTESIAN_POINT ( 'NONE',  ( 20.92131311655350245, -1.145359114192535888, -15.19233952661473097 ) ) ;
#8861=CARTESIAN_POINT ( 'NONE',  ( 19.80084360436371682, 0.3372488075446856692, -14.31343108369374484 ) ) ;
#8880=ORIENTED_EDGE ( 'NONE', *, *, #1863, .F. ) ;
#8887=( GEOMETRIC_REPRESENTATION_CONTEXT ( 3 ) GLOBAL_UNCERTAINTY_ASSIGNED_CONTEXT ( ( #20948 ) ) GLOBAL_UNIT_ASSIGNED_CONTEXT ( ( #3435, #15069, #13961 ) ) REPRESENTATION_CONTEXT ( 'NONE', 'WORKASPACE' ) );
#8889=CARTESIAN_POINT ( 'NONE',  ( 19.58772840857323772, -1.669332001046654801, -14.30030513082031618 ) ) ;
#8895=ORIENTED_EDGE ( 'NONE', *, *, #9400, .F. ) ;
#8923=CARTESIAN_POINT ( 'NONE',  ( 13.63956567280660614, -6.673707092738088598, -15.35198154347669508 ) ) ;
#8932=CARTESIAN_POINT ( 'NONE',  ( 14.54968198082151609, -8.672570558313584144, -15.03874522469199171 ) ) ;
#8976=CARTESIAN_POINT ( 'NONE',  ( 20.94353291967679453, -2.672331840313235674, -13.89923075121346230 ) ) ;
#8982=CARTESIAN_POINT ( 'NONE',  ( 11.26949333533593922, -4.616615725918594038, -15.82154907933577448 ) ) ;
#9000=CARTESIAN_POINT ( 'NONE',  ( 19.80556909575297908, -1.573965866645507861, -15.31865534271369711 ) ) ;
#9001=CARTESIAN_POINT ( 'NONE',  ( 16.92565045872677487, 0.9375092998980070202, -15.17115336936947934 ) ) ;
#9018=CARTESIAN_POINT ( 'NONE',  ( 14.81625953204187596, -7.424720918027729155, -15.06137846235305844 ) ) ;
#9037=CARTESIAN_POINT ( 'NONE',  ( 14.20533558566156884, -7.867031480749381522, -15.79333615885272835 ) ) ;
#9050=CARTESIAN_POINT ( 'NONE',  ( 11.81489480681374715, -4.423560566030090513, -15.68132100509055782 ) ) ;
#9079=FACE_OUTER_BOUND ( 'NONE', #3940, .T. ) ;
#9080=CARTESIAN_POINT ( 'NONE',  ( 14.91885465629891172, 2.197622263519783736, -15.77636844865548582 ) ) ;
#9093=DIRECTION ( 'NONE',  ( -0.3482992169606098365, 0.9330960544336215357, -0.08955115110948595747 ) ) ;
#9101=ADVANCED_FACE ( 'NONE', ( #394 ), #17197, .T. ) ;
#9102=CARTESIAN_POINT ( 'NONE',  ( 18.38685979067734166, 0.1402437363902317435, -14.71391125517748222 ) ) ;
#9122=CARTESIAN_POINT ( 'NONE',  ( 19.35098353498187507, 0.3056836383201791962, -15.04733789981717251 ) ) ;
#9125=CARTESIAN_POINT ( 'NONE',  ( 20.59926559563684378, -3.336837234538238217, -15.67345047278095471 ) ) ;
#9188=CARTESIAN_POINT ( 'NONE',  ( 19.44826403579765284, 0.7519677144109497835, -14.42437082291665362 ) ) ;
#9199=ORIENTED_EDGE ( 'NONE', *, *, #10471, .T. ) ;
#9204=CARTESIAN_POINT ( 'NONE',  ( 17.97854127242967337, -8.300061438778795875, -14.56394595263420477 ) ) ;
#9212=DIRECTION ( 'NONE',  ( -0.3482992169606098365, 0.9330960544336215357, -0.08955115110948595747 ) ) ;
#9215=DIRECTION ( 'NONE',  ( -0.1132953773954069598, 0.7241889112991808375, -0.6802312681817410667 ) ) ;
#9235=CARTESIAN_POINT ( 'NONE',  ( 19.38375428936542377, 0.2020908859931673240, -15.04237192290629110 ) ) ;
#9236=CARTESIAN_POINT ( 'NONE',  ( 16.94501325483539844, 1.212346912392092024, -15.11607461051017331 ) ) ;
#9259=VERTEX_POINT ( 'NONE', #12127 ) ;
#9318=APPLICATION_CONTEXT ( 'automotive_design' ) ;
#9347=CARTESIAN_POINT ( 'NONE',  ( 17.43388704644383580, -7.135208455246296211, -14.50876463681930773 ) ) ;
#9376=FACE_OUTER_BOUND ( 'NONE', #941, .T. ) ;
#9400=EDGE_CURVE ( 'NONE', #9259, #20548, #12046, .T. ) ;
#9414=CARTESIAN_POINT ( 'NONE',  ( 11.67127651341588113, -6.514806905098483369, -15.79013620009136076 ) ) ;
#9445=CARTESIAN_POINT ( 'NONE',  ( 20.24903775639316805, -5.937233424764036371, -13.47572151283328878 ) ) ;
#9453=CARTESIAN_POINT ( 'NONE',  ( 20.20304770538988137, -1.338751018026005379, -14.76265918450644854 ) ) ;
#9459=CARTESIAN_POINT ( 'NONE',  ( 20.88124149777159388, -1.145906272312793517, -15.04208939847202409 ) ) ;
#9487=CARTESIAN_POINT ( 'NONE',  ( 8.231104565076774904, 2.698862664129421329, -16.60274868773344537 ) ) ;
#9517=CARTESIAN_POINT ( 'NONE',  ( 14.65261474522852936, -8.323537342180904020, -15.15547592125267151 ) ) ;
#9554=CARTESIAN_POINT ( 'NONE',  ( 14.49583489321334007, -8.530823778528098700, -14.71411849925045523 ) ) ;
#9561=CARTESIAN_POINT ( 'NONE',  ( 19.62005440932008682, -0.3128815169959983655, -14.95834899907133142 ) ) ;
#9589=LINE ( 'NONE', #14603, #5358 ) ;
#9630=CARTESIAN_POINT ( 'NONE',  ( 14.60635709262053439, -8.313957965053235810, -15.16560502254627174 ) ) ;
#9656=CARTESIAN_POINT ( 'NONE',  ( 20.14654830070027813, -6.335923874353329488, -15.19130692721172515 ) ) ;
#9664=CARTESIAN_POINT ( 'NONE',  ( 11.72582454026615828, -4.501321389889026747, -15.56411338575258974 ) ) ;
#9670=CARTESIAN_POINT ( 'NONE',  ( 19.39617148027078741, 0.1681879138596751311, -15.03931347124663453 ) ) ;
#9671=EDGE_CURVE ( 'NONE', #13654, #14268, #16535, .T. ) ;
#9675=CARTESIAN_POINT ( 'NONE',  ( 19.75185127208544600, 0.1555953079926848670, -15.00720622995094189 ) ) ;
#9681=CARTESIAN_POINT ( 'NONE',  ( 19.13386765903375775, -5.735230366684957559, -15.44418781123290429 ) ) ;
#9689=CARTESIAN_POINT ( 'NONE',  ( 17.93242123830337320, -8.292540772221606460, -14.39788784616911776 ) ) ;
#9735=CARTESIAN_POINT ( 'NONE',  ( 20.88318715027774530, -3.948290930238875784, -13.86799592610689658 ) ) ;
#9737=ORIENTED_EDGE ( 'NONE', *, *, #6648, .F. ) ;
#9768=CARTESIAN_POINT ( 'NONE',  ( 20.01377712881487980, -2.741521743599813821, -13.99508467333011907 ) ) ;
#9773=EDGE_CURVE ( 'NONE', #624, #13225, #1910, .T. ) ;
#9834=CARTESIAN_POINT ( 'NONE',  ( 18.23145731651337087, -7.767129607868482388, -14.37336575840138231 ) ) ;
#9868=CARTESIAN_POINT ( 'NONE',  ( 19.42376837693508307, -5.426032880614602760, -13.68790637948557887 ) ) ;
#9878=CARTESIAN_POINT ( 'NONE',  ( 11.36393682984004450, -4.708245059028417501, -16.48153251965310062 ) ) ;
#9885=CARTESIAN_POINT ( 'NONE',  ( 18.94865055687374422, -5.956368045175373993, -15.47817826132612140 ) ) ;
#9900=ORIENTED_EDGE ( 'NONE', *, *, #3460, .T. ) ;
#9984=CARTESIAN_POINT ( 'NONE',  ( 16.99218898555291446, -8.338783895011660618, -15.86074989063387264 ) ) ;
#9995=CARTESIAN_POINT ( 'NONE',  ( 11.51778461937661291, -4.547966530721023304, -15.27913115286716206 ) ) ;
#10011=CARTESIAN_POINT ( 'NONE',  ( 17.25519468990899341, -7.034179569086526307, -15.81717762532307958 ) ) ;
#10033=TOROIDAL_SURFACE ( 'NONE', #12881, 3.174999999999999822, 0.5953125000000000222 ) ;
#10067=CARTESIAN_POINT ( 'NONE',  ( 10.72409186464205355, -4.809670885807086016, -15.96177715662992824 ) ) ;
#10091=CARTESIAN_POINT ( 'NONE',  ( 11.17185072860094763, -5.218912923018368843, -17.09259198936415913 ) ) ;
#10100=CARTESIAN_POINT ( 'NONE',  ( 20.07182034886884381, -2.730729751928062665, -13.64168985034137549 ) ) ;
#10107=CARTESIAN_POINT ( 'NONE',  ( 20.39211608684103538, -6.633859764968358164, -15.26783537666067403 ) ) ;
#10114=CARTESIAN_POINT ( 'NONE',  ( 11.98346169735263445, -2.082869424899609800, -16.75639176224798277 ) ) ;
#10145=CARTESIAN_POINT ( 'NONE',  ( 19.79612130048327145, -2.801990398175632002, -14.19231935140637724 ) ) ;
#10159=EDGE_CURVE ( 'NONE', #6378, #5048, #16334, .T. ) ;
#10181=PRODUCT_DEFINITION_FORMATION_WITH_SPECIFIED_SOURCE ( 'ANY', '', #19193, .NOT_KNOWN. ) ;
#10193=CARTESIAN_POINT ( 'NONE',  ( 15.22903305875954594, -8.380302064858637934, -16.24791865429935100 ) ) ;
#10203=CARTESIAN_POINT ( 'NONE',  ( 12.36433962874629877, -0.5403542521652121566, -16.63866349071987827 ) ) ;
#10220=CARTESIAN_POINT ( 'NONE',  ( 12.34662851096885916, -4.975191070769994006, -16.80281937503197298 ) ) ;
#10221=CARTESIAN_POINT ( 'NONE',  ( 10.85253788098002836, -4.717387943497917568, -15.38032343689423875 ) ) ;
#10253=CARTESIAN_POINT ( 'NONE',  ( 13.84999724918104391, -6.798182784255816458, -15.30952765826574513 ) ) ;
#10258=DIRECTION ( 'NONE',  ( -0.3140771401027084853, 0.9459569826691583971, -0.08075231887918270235 ) ) ;
#10298=ADVANCED_FACE ( 'NONE', ( #12690 ), #16234, .T. ) ;
#10310=CARTESIAN_POINT ( 'NONE',  ( 10.82835441204896298, -1.966650465303993567, -17.05962226904667389 ) ) ;
#10323=CIRCLE ( 'NONE', #8208, 3.770312499999998845 ) ;
#10324=DIRECTION ( 'NONE',  ( 0.4128958666089267981, -0.5884034904305870395, -0.6951966166390379787 ) ) ;
#10327=CARTESIAN_POINT ( 'NONE',  ( 20.07493000556766205, 0.4717600457865012142, -14.72462693936004285 ) ) ;
#10339=CARTESIAN_POINT ( 'NONE',  ( 15.99064506707870414, 1.097848371653701083, -15.45815286304121727 ) ) ;
#10341=ORIENTED_EDGE ( 'NONE', *, *, #9773, .T. ) ;
#10372=CARTESIAN_POINT ( 'NONE',  ( 16.69192786310252785, -7.118735165633143680, -14.71864076686690126 ) ) ;
#10422=CARTESIAN_POINT ( 'NONE',  ( 20.23867309534036707, -1.248700931907035239, -14.75477345577187371 ) ) ;
#10429=DIRECTION ( 'NONE',  ( -0.9161599507719021540, -0.3242921320961419940, -0.2355537256384720723 ) ) ;
#10436=VERTEX_POINT ( 'NONE', #232 ) ;
#10449=CARTESIAN_POINT ( 'NONE',  ( 18.00500580558605890, 0.4330974563432516966, -14.83538992815904400 ) ) ;
#10471=EDGE_CURVE ( 'NONE', #13225, #13907, #17595, .T. ) ;
#10478=CARTESIAN_POINT ( 'NONE',  ( 16.92682437108570426, -7.051316376102997552, -14.66989665197142578 ) ) ;
#10486=CARTESIAN_POINT ( 'NONE',  ( 17.55130215754536493, -8.551187338024273998, -15.76935921083538084 ) ) ;
#10528=CARTESIAN_POINT ( 'NONE',  ( 18.53801154572697385, 1.494989082069840824, -14.70250965503444540 ) ) ;
#10551=CARTESIAN_POINT ( 'NONE',  ( 18.91132178901277072, -0.4204008045333961219, -14.54213590646165422 ) ) ;
#10553=CARTESIAN_POINT ( 'NONE',  ( 10.97846818458738127, -4.667157448163489875, -15.28170016135478804 ) ) ;
#10582=EDGE_LOOP ( 'NONE', ( #4506, #16127, #18334, #18219 ) ) ;
#10588=CARTESIAN_POINT ( 'NONE',  ( 14.07100346269973201, -6.903878524309663867, -15.26435492765976321 ) ) ;
#10596=CARTESIAN_POINT ( 'NONE',  ( 20.46393712135811072, -0.2355988221118890391, -15.20378812335061092 ) ) ;
#10603=VECTOR ( 'NONE', #11863, 1000.000000000000000 ) ;
#10641=DIRECTION ( 'NONE',  ( -0.2490110332224855227, 0.000000000000000000, 0.9685006480810791629 ) ) ;
#10645=CARTESIAN_POINT ( 'NONE',  ( 20.95242871594548362, -3.348541484849226535, -13.87224525169349043 ) ) ;
#10664=CARTESIAN_POINT ( 'NONE',  ( 21.56733905798141393, -3.402205227929565812, -14.90816191201569474 ) ) ;
#10672=CARTESIAN_POINT ( 'NONE',  ( 15.75244874201758094, 1.099573029051923667, -15.53104562322756088 ) ) ;
#10691=CARTESIAN_POINT ( 'NONE',  ( 19.58283533066354565, 0.2704557082564330583, -14.92202265744526990 ) ) ;
#10692=CARTESIAN_POINT ( 'NONE',  ( 20.34020935552985065, -3.329038851323427917, -15.20636776770394683 ) ) ;
#10706=ORIENTED_EDGE ( 'NONE', *, *, #3973, .T. ) ;
#10712=CARTESIAN_POINT ( 'NONE',  ( 17.20754637584470714, -7.943092760107163919, -15.14184226529886246 ) ) ;
#10728=CARTESIAN_POINT ( 'NONE',  ( 11.68644878885729277, -4.515843508674393547, -16.26277472245715927 ) ) ;
#10757=CARTESIAN_POINT ( 'NONE',  ( 19.74951347795774481, 0.4024288987411958618, -14.32971591649493170 ) ) ;
#10780=CARTESIAN_POINT ( 'NONE',  ( 19.29498493895778211, -0.9933881662693676562, -14.41052274056791305 ) ) ;
#10799=CARTESIAN_POINT ( 'NONE',  ( 19.34116629174159030, 0.4109076020908116189, -15.03439639987123755 ) ) ;
#10800=CARTESIAN_POINT ( 'NONE',  ( 17.18860471232197540, -7.336512682313781397, -15.77586843043927267 ) ) ;
#10827=ORIENTED_EDGE ( 'NONE', *, *, #13387, .F. ) ;
#10860=CARTESIAN_POINT ( 'NONE',  ( 20.05460976202589407, -0.006649262762246921366, -14.23230800686313735 ) ) ;
#10874=CARTESIAN_POINT ( 'NONE',  ( 21.03649535373696722, -1.171894805719116084, -15.12491633086513687 ) ) ;
#10884=ORIENTED_EDGE ( 'NONE', *, *, #1308, .T. ) ;
#10899=CARTESIAN_POINT ( 'NONE',  ( 19.34511922692029984, 0.3276742896394955196, -15.04744788783380827 ) ) ;
#10904=CARTESIAN_POINT ( 'NONE',  ( 11.60664369415897568, -3.109370887057594235, -16.86713491734067460 ) ) ;
#10914=CARTESIAN_POINT ( 'NONE',  ( 19.67909734877197891, 0.1298811790940870847, -14.89708569419555317 ) ) ;
#10918=CARTESIAN_POINT ( 'NONE',  ( 11.44554379814851508, -6.402327797446566215, -17.01165796439540756 ) ) ;
#10939=VECTOR ( 'NONE', #13766, 1000.000000000000000 ) ;
#10967=CARTESIAN_POINT ( 'NONE',  ( 19.64230669971109222, 0.5287862484321461665, -14.36345453931188665 ) ) ;
#11008=AXIS2_PLACEMENT_3D ( 'NONE', #1442, #4662, #21678 ) ;
#11014=CARTESIAN_POINT ( 'NONE',  ( 19.42050984830941829, -5.834154119974274799, -15.51764488770388972 ) ) ;
#11083=CARTESIAN_POINT ( 'NONE',  ( 14.89546171155516063, -8.373827889660200086, -15.10229938975829178 ) ) ;
#11104=LINE ( 'NONE', #12449, #14524 ) ;
#11114=CARTESIAN_POINT ( 'NONE',  ( 17.12871318600645409, 2.301163489826294484, -14.63919962258086827 ) ) ;
#11122=CARTESIAN_POINT ( 'NONE',  ( 19.98142615554668566, -0.9834789709510379785, -14.83023175912481051 ) ) ;
#11123=CARTESIAN_POINT ( 'NONE',  ( 19.93414139600567125, -1.593704270021353953, -15.40834236525699730 ) ) ;
#11127=CARTESIAN_POINT ( 'NONE',  ( 20.23508918937977796, -1.359453322992689506, -14.75410208910826704 ) ) ;
#11139=CARTESIAN_POINT ( 'NONE',  ( 17.52996087073869447, -8.549669343631473239, -15.68810240790472577 ) ) ;
#11147=SHAPE_REPRESENTATION ( 'Handle Pawl Torsion Spring', ( #2234 ), #4182 ) ;
#11149=EDGE_CURVE ( 'NONE', #13907, #13654, #7718, .T. ) ;
#11185=CARTESIAN_POINT ( 'NONE',  ( 11.77191967066123723, -6.633846379865024012, -15.76999337786026345 ) ) ;
#11208=CARTESIAN_POINT ( 'NONE',  ( 20.53156541068710439, -1.359447366214681985, -15.90722246059563361 ) ) ;
#11218=CARTESIAN_POINT ( 'NONE',  ( 20.80998580648388341, -1.217322788665459177, -14.73620959842755695 ) ) ;
#11224=CARTESIAN_POINT ( 'NONE',  ( 20.00345035822784467, -1.023028193093147076, -14.82316847688469785 ) ) ;
#11227=CARTESIAN_POINT ( 'NONE',  ( 12.11904762564861926, -6.033546283575153879, -17.57169469594360578 ) ) ;
#11232=CARTESIAN_POINT ( 'NONE',  ( 20.07818426912813337, -3.465737206707578011, -15.31859466601284403 ) ) ;
#11233=CARTESIAN_POINT ( 'NONE',  ( 13.99260895880537525, 15.36419388438619649, -16.35910307397442054 ) ) ;
#11240=CARTESIAN_POINT ( 'NONE',  ( 21.27104401621292595, -2.646375628860768270, -13.78030298333726478 ) ) ;
#11290=CARTESIAN_POINT ( 'NONE',  ( 20.65970833833902986, -4.825822034318000497, -13.89237661239871358 ) ) ;
#11296=VERTEX_POINT ( 'NONE', #10067 ) ;
#11329=CARTESIAN_POINT ( 'NONE',  ( 19.37933662139949931, -5.924303267933944461, -14.90337022717902471 ) ) ;
#11334=( NAMED_UNIT ( * ) PLANE_ANGLE_UNIT ( ) SI_UNIT ( $, .RADIAN. ) );
#11338=CARTESIAN_POINT ( 'NONE',  ( 20.13639834117197935, -1.248927570271565646, -14.78218852182811993 ) ) ;
#11340=CARTESIAN_POINT ( 'NONE',  ( 19.33254070244220557, -0.1605694297987687869, -14.91550252399787091 ) ) ;
#11356=CARTESIAN_POINT ( 'NONE',  ( 11.33405156777011236, 0.1799087130929279132, -16.79951585329149921 ) ) ;
#11371=FACE_OUTER_BOUND ( 'NONE', #2778, .T. ) ;
#11376=AXIS2_PLACEMENT_3D ( 'NONE', #2812, #11536, #7785 ) ;
#11380=CARTESIAN_POINT ( 'NONE',  ( 11.97174136233939556, 21.25996874134203551, -17.62449286037261942 ) ) ;
#11398=AXIS2_PLACEMENT_3D ( 'NONE', #681, #17499, #10641 ) ;
#11408=CARTESIAN_POINT ( 'NONE',  ( 16.85565294364209876, -8.302906301136502520, -14.67196852948350561 ) ) ;
#11436=CARTESIAN_POINT ( 'NONE',  ( 19.93266995306398925, -6.610076642783412559, -15.23350694284797235 ) ) ;
#11445=CARTESIAN_POINT ( 'NONE',  ( 17.20909397020470166, -7.334998182188638083, -15.85734429837840764 ) ) ;
#11507=CARTESIAN_POINT ( 'NONE',  ( 17.58883026422746454, -8.071787399390844442, -14.51212895374598055 ) ) ;
#11536=DIRECTION ( 'NONE',  ( -0.3482992169606098920, 0.9330960544336215357, -0.08955115110948595747 ) ) ;
#11538=CARTESIAN_POINT ( 'NONE',  ( 21.58408671149279812, -3.402206684524639702, -14.97329867675111537 ) ) ;
#11545=CARTESIAN_POINT ( 'NONE',  ( 19.94507429925241127, -1.548276246954950697, -14.95858684565857644 ) ) ;
#11562=CARTESIAN_POINT ( 'NONE',  ( 14.99032816781414290, -7.116660944607684058, -16.28946189193466054 ) ) ;
#11586=DIRECTION ( 'NONE',  ( 0.3697464814795229371, -0.9291326812858928808, 0.000000000000000000 ) ) ;
#11653=CARTESIAN_POINT ( 'NONE',  ( 12.12836021491582983, -0.4634883892451792109, -16.16564750685157748 ) ) ;
#11661=AXIS2_PLACEMENT_3D ( 'NONE', #6482, #13449, #3059 ) ;
#11668=CARTESIAN_POINT ( 'NONE',  ( 11.87797320575361049, -2.913634519652867461, -16.82300781167370829 ) ) ;
#11669=CARTESIAN_POINT ( 'NONE',  ( 14.28908772023590323, 15.36419388438619649, -17.51222415809595390 ) ) ;
#11761=CARTESIAN_POINT ( 'NONE',  ( 14.27942466917048492, -8.136872695340121808, -16.45546583691613662 ) ) ;
#11771=CARTESIAN_POINT ( 'NONE',  ( 12.31258714455350045, -6.210927838223190278, -15.15504894760450227 ) ) ;
#11784=CARTESIAN_POINT ( 'NONE',  ( 14.23877267092113108, -6.845582297732573984, -16.44448175767178100 ) ) ;
#11787=ORIENTED_EDGE ( 'NONE', *, *, #6028, .F. ) ;
#11820=CARTESIAN_POINT ( 'NONE',  ( 19.72286286404087363, -3.871483444068603230, -14.16070975014500632 ) ) ;
#11863=DIRECTION ( 'NONE',  ( -0.3140771401027084853, 0.9459569826691583971, -0.08075231887918268847 ) ) ;
#11865=CARTESIAN_POINT ( 'NONE',  ( 10.72442325415146946, -2.948066920625321607, -17.12250937314169974 ) ) ;
#11888=CARTESIAN_POINT ( 'NONE',  ( 16.78551053486653544, -7.162656031619696329, -15.91463781719514081 ) ) ;
#11907=CARTESIAN_POINT ( 'NONE',  ( 20.22951472560300346, -1.344520626714845069, -14.75553331646387711 ) ) ;
#11912=VERTEX_POINT ( 'NONE', #10914 ) ;
#11914=DIRECTION ( 'NONE',  ( 0.9037041334408600912, 0.3596272420165190775, 0.2323512126103423614 ) ) ;
#11918=CARTESIAN_POINT ( 'NONE',  ( 18.74736864250175472, -5.850096548006167296, -14.30666788301311954 ) ) ;
#11966=CARTESIAN_POINT ( 'NONE',  ( 20.22718371673215287, -1.176379440366829954, -14.75900186987939300 ) ) ;
#11970=CARTESIAN_POINT ( 'NONE',  ( 10.72528277947465014, -3.117068478670475429, -17.12846307055972872 ) ) ;
#12018=AXIS2_PLACEMENT_3D ( 'NONE', #14231, #9215, #7572 ) ;
#12028=CARTESIAN_POINT ( 'NONE',  ( 13.42913409643213107, -6.549231401220326987, -15.39443542868764503 ) ) ;
#12046=CIRCLE ( 'NONE', #15599, 0.5953125000000005773 ) ;
#12058=SURFACE_STYLE_FILL_AREA ( #1654 ) ;
#12060=ORIENTED_EDGE ( 'NONE', *, *, #16028, .F. ) ;
#12089=CARTESIAN_POINT ( 'NONE',  ( 10.73605050800646943, -2.562123915646048022, -17.10540653823293766 ) ) ;
#12115=CARTESIAN_POINT ( 'NONE',  ( 16.88793093518696509, 0.9484654469177136171, -15.18277371644746765 ) ) ;
#12127=CARTESIAN_POINT ( 'NONE',  ( 12.91059077353605211, 21.25996874134203907, -21.27604296009081253 ) ) ;
#12136=FACE_BOUND ( 'NONE', #16640, .T. ) ;
#12149=CARTESIAN_POINT ( 'NONE',  ( 14.88133261977736232, -7.156567809876259290, -15.09667001033014166 ) ) ;
#12164=AXIS2_PLACEMENT_3D ( 'NONE', #5896, #9212, #20944 ) ;
#12196=CARTESIAN_POINT ( 'NONE',  ( 19.87209107541814035, -0.1962630820641820817, -14.85150087166202226 ) ) ;
#12200=CARTESIAN_POINT ( 'NONE',  ( 13.04431081968415462, 1.431559631576304170, -16.33551417402710726 ) ) ;
#12215=CARTESIAN_POINT ( 'NONE',  ( 21.61819370792156292, -3.402680683349632140, -15.07300270223215222 ) ) ;
#12222=CARTESIAN_POINT ( 'NONE',  ( 18.72819589094305570, -0.2033655786179353053, -14.60285019604222967 ) ) ;
#12223=CARTESIAN_POINT ( 'NONE',  ( 11.77608582838452023, -4.423560565762836738, -15.53037780770169363 ) ) ;
#12246=ORIENTED_EDGE ( 'NONE', *, *, #16028, .T. ) ;
#12252=CARTESIAN_POINT ( 'NONE',  ( 12.53020504515603761, -5.716024679458021396, -15.56730839992324356 ) ) ;
#12262=CARTESIAN_POINT ( 'NONE',  ( 20.32304652538368828, -6.633862778167403107, -14.99920447863399353 ) ) ;
#12298=CARTESIAN_POINT ( 'NONE',  ( 20.23296939222377233, -1.209661760518722762, -14.75693070578325106 ) ) ;
#12302=CARTESIAN_POINT ( 'NONE',  ( 20.76278067970291374, -1.556605016331053637, -13.98716170710216211 ) ) ;
#12310=CARTESIAN_POINT ( 'NONE',  ( 14.39766489109863734, 1.100710950241990504, -15.99547158540225489 ) ) ;
#12317=CARTESIAN_POINT ( 'NONE',  ( 20.48375339570359444, -0.2396799350905462478, -15.30716636276063447 ) ) ;
#12325=CARTESIAN_POINT ( 'NONE',  ( 12.20717034251990540, -1.379848799635395640, -16.66392367771780414 ) ) ;
#12348=CARTESIAN_POINT ( 'NONE',  ( 12.39411805528681576, -0.5459497824433883206, -16.72217961216554372 ) ) ;
#12371=CARTESIAN_POINT ( 'NONE',  ( 20.06905745580504785, 0.5585409057930410537, -14.27919157916436532 ) ) ;
#12389=VERTEX_POINT ( 'NONE', #20460 ) ;
#12393=CARTESIAN_POINT ( 'NONE',  ( 20.67155644328900621, -1.303699069785051456, -15.87085131396228199 ) ) ;
#12421=CARTESIAN_POINT ( 'NONE',  ( 20.96272718584998529, -3.045802774718411321, -13.88062344517622826 ) ) ;
#12440=CARTESIAN_POINT ( 'NONE',  ( 10.38009686120726904, -3.119983079838188011, -17.18249216028544524 ) ) ;
#12447=CARTESIAN_POINT ( 'NONE',  ( 20.09375723660039270, -1.415681770550045515, -14.79025032679060381 ) ) ;
#12448=CARTESIAN_POINT ( 'NONE',  ( 16.22686663214561520, 1.074243784483314146, -15.38576787205390062 ) ) ;
#12449=CARTESIAN_POINT ( 'NONE',  ( 20.23508736156870569, -1.359449706705495364, -14.75410053729980397 ) ) ;
#12466=CARTESIAN_POINT ( 'NONE',  ( 19.37359715633457569, 0.4386801721828464951, -15.00800319500494950 ) ) ;
#12468=CARTESIAN_POINT ( 'NONE',  ( 20.17739840222535719, -1.548276265051773404, -15.86218595987928026 ) ) ;
#12499=PRODUCT_DEFINITION_SHAPE ( 'NONE', 'NONE',  #5596 ) ;
#12535=CARTESIAN_POINT ( 'NONE',  ( 18.78053651718387229, 1.329081106205024954, -14.62912815047282855 ) ) ;
#12559=CARTESIAN_POINT ( 'NONE',  ( 14.58714708142341721, 0.8861103173364321961, -15.88890669882432682 ) ) ;
#12577=CARTESIAN_POINT ( 'NONE',  ( 19.38085053746658915, -5.840261935552881312, -15.33262441706652268 ) ) ;
#12580=CARTESIAN_POINT ( 'NONE',  ( 20.68769545271989330, -1.192153677757474384, -14.77120002427500900 ) ) ;
#12594=B_SPLINE_CURVE_WITH_KNOTS ( 'NONE', 3,
 ( #1783, #16832, #13642, #10422, #18588, #5540, #12298, #19026, #11966, #3455, #18918, #3678, #16, #8528, #17270, #1673, #17163, #20572, #8413, #351, #5210, #6883, #15189, #8742, #5431, #12196, #2116, #5113, #15308, #15641, #15523, #472, #6766, #20238, #16933, #131, #20342, #8644 ),
 .UNSPECIFIED., .F., .F.,
 ( 4, 2, 2, 2, 1, 1, 2, 2, 1, 2, 2, 2, 2, 1, 2, 2, 2, 2, 2, 1, 1, 4 ),
 ( 5.534983508193036528E-06, 0.04939775905433628489, 0.06174581507204322806, 0.06791984308089690781, 0.07409387108975057368, 0.09878998312516618086, 0.1234860951605817880, 0.1296601231694354261, 0.1358341511782890920, 0.1481822071959962572, 0.1975744312668257507, 0.2469666553376552443, 0.2593147113553626038, 0.2716627673730700465, 0.2963588794084849320, 0.3457511034793138704, 0.3704472155147284784, 0.3735342295191548811, 0.3750777365213670000, 0.3766212435235791745, 0.3827952715324290933, 0.3951433275501288200 ),
 .UNSPECIFIED. ) ;
#12604=DIRECTION ( 'NONE',  ( -0.4128958666089269647, 0.5884034904305883718, 0.6951966166390366464 ) ) ;
#12606=CARTESIAN_POINT ( 'NONE',  ( 20.53156541068710439, -1.359447366214681985, -15.90722246059563361 ) ) ;
#12635=DIRECTION ( 'NONE',  ( -0.3140771401027084853, 0.9459569826691583971, -0.08075231887918268847 ) ) ;
#12639=CARTESIAN_POINT ( 'NONE',  ( 18.28386440432367621, 1.638836122736962331, -14.77887936977548300 ) ) ;
#12665=CARTESIAN_POINT ( 'NONE',  ( 14.59864429982308032, -8.662966625467099391, -15.22137380051930045 ) ) ;
#12680=CARTESIAN_POINT ( 'NONE',  ( 11.66912023571120827, -3.656888143346838316, -15.82494830968131438 ) ) ;
#12690=FACE_OUTER_BOUND ( 'NONE', #432, .T. ) ;
#12693=CARTESIAN_POINT ( 'NONE',  ( 17.27120983696573120, 2.432768651782924785, -15.04950751273090148 ) ) ;
#12750=CARTESIAN_POINT ( 'NONE',  ( 12.40265734679424092, -7.252961835381453781, -15.64046151589976930 ) ) ;
#12777=CARTESIAN_POINT ( 'NONE',  ( 20.39032348261012118, -1.415670249624013666, -15.94372942033169593 ) ) ;
#12783=CARTESIAN_POINT ( 'NONE',  ( 10.66005185129409938, -4.911957254796272210, -16.03335128564671308 ) ) ;
#12789=CARTESIAN_POINT ( 'NONE',  ( 10.40440438601274487, -3.118828651999451473, -16.72929749093172092 ) ) ;
#12799=CARTESIAN_POINT ( 'NONE',  ( 20.04236263901815462, -1.092632170845033057, -14.81078003435047563 ) ) ;
#12800=TOROIDAL_SURFACE ( 'NONE', #17017, 3.174999999999999822, 0.5953125000000000222 ) ;
#12801=FACE_OUTER_BOUND ( 'NONE', #21100, .T. ) ;
#12863=CARTESIAN_POINT ( 'NONE',  ( 11.81489480602983733, -4.423560566030109165, -15.68132100204162249 ) ) ;
#12867=CARTESIAN_POINT ( 'NONE',  ( 17.85888992747382886, -7.950010299323909457, -14.45371996643464918 ) ) ;
#12881=AXIS2_PLACEMENT_3D ( 'NONE', #19552, #4419, #16144 ) ;
#12890=CARTESIAN_POINT ( 'NONE',  ( 20.64792629172051974, -5.531186785911284431, -15.09723995909050309 ) ) ;
#12903=CARTESIAN_POINT ( 'NONE',  ( 17.51061561465282068, -8.559080621069766082, -15.60190410038134878 ) ) ;
#12918=CARTESIAN_POINT ( 'NONE',  ( 20.03282866373563209, -3.767791603764007125, -15.31592657159819204 ) ) ;
#12974=CARTESIAN_POINT ( 'NONE',  ( 11.08661322212816458, -5.636319538762833758, -15.90164728704758801 ) ) ;
#12988=B_SPLINE_CURVE_WITH_KNOTS ( 'NONE', 3,
 ( #2594, #18969, #7889, #12777, #4473, #11208 ),
 .UNSPECIFIED., .F., .F.,
 ( 4, 1, 1, 4 ),
 ( 0.000000000000000000, 0.2500007535536921122, 0.5000000202745886746, 0.5007142149769521211 ),
 .UNSPECIFIED. ) ;
#12999=CARTESIAN_POINT ( 'NONE',  ( 21.15028308705900884, -4.113433257334989435, -15.02320902816535053 ) ) ;
#13001=AXIS2_PLACEMENT_3D ( 'NONE', #2730, #14039, #20744 ) ;
#13011=CARTESIAN_POINT ( 'NONE',  ( 17.94914520215607823, -8.292551780608357959, -14.46302984805736003 ) ) ;
#13025=CARTESIAN_POINT ( 'NONE',  ( 19.98943338725409546, -4.012182358950986405, -15.31543382922598262 ) ) ;
#13050=ORIENTED_EDGE ( 'NONE', *, *, #20215, .T. ) ;
#13075=DIRECTION ( 'NONE',  ( 0.4128958666089267981, -0.5884034904305870395, -0.6951966166390379787 ) ) ;
#13084=VERTEX_POINT ( 'NONE', #11233 ) ;
#13106=CARTESIAN_POINT ( 'NONE',  ( 12.61411201210553124, 21.25996874134203907, -20.12292187596927562 ) ) ;
#13117=CARTESIAN_POINT ( 'NONE',  ( 14.57805970825261355, -7.268432535603025713, -16.41340505930001115 ) ) ;
#13127=CIRCLE ( 'NONE', #14542, 0.5953125000000000222 ) ;
#13192=CARTESIAN_POINT ( 'NONE',  ( 11.57594508772183417, -6.391478118055172075, -15.80891331407196354 ) ) ;
#13216=CARTESIAN_POINT ( 'NONE',  ( 21.25318714072498594, -3.068702901631692459, -15.03512189218206707 ) ) ;
#13225=VERTEX_POINT ( 'NONE', #11669 ) ;
#13229=CARTESIAN_POINT ( 'NONE',  ( 19.42330635861384991, 0.1555817663055659994, -13.72932059668182170 ) ) ;
#13237=CARTESIAN_POINT ( 'NONE',  ( 20.22083624039512273, -1.348948031050671847, -14.75776464959390211 ) ) ;
#13239=CARTESIAN_POINT ( 'NONE',  ( 11.22134872449618825, -3.741537362231782460, -16.47805867944655489 ) ) ;
#13245=CARTESIAN_POINT ( 'NONE',  ( 12.54707462758905834, -5.336976515233779139, -16.77073826699180259 ) ) ;
#13246=ADVANCED_FACE ( 'NONE', ( #8126 ), #6690, .T. ) ;
#13261=B_SPLINE_CURVE_WITH_KNOTS ( 'NONE', 3,
 ( #14990, #14769, #19819, #16314, #21705, #14874, #6453, #13216, #4802, #21266, #4578, #13323, #3034, #12999, #19930, #7781, #4692, #14547, #12890, #21372, #6227, #2930, #9656, #21476, #6333, #11436, #18181, #5117, #17166, #15092, #18814, #134, #3458, #16835, #8647, #13873, #2006, #8746, #5435, #5005, #9984, #15527, #6886, #17053, #21805, #5322, #10193, #356, #15311, #3681, #1580, #11761, #1788, #13646, #18490, #8321, #7104, #18376, #13756, #13535, #15194, #3247, #16740, #16937, #6659, #13419, #20346, #20129, #8531, #3363, #10091, #6769, #1677, #8417, #20452, #5214, #19, #20242, #11970, #18701, #11865, #18591, #12089, #3569, #10310, #1899, #15421, #247, #6985, #14312, #17720, #7549, #20917, #21127, #21029, #19149, #2121, #685, #4118, #910, #2350, #12200, #5779, #7651, #2571, #2238, #14412, #4015, #9080, #3792, #17398, #7430, #17274, #5544, #18922, #5875, #476, #5662, #14090, #14203, #19259, #20795, #15645, #12639, #10528, #12535, #7230, #802, #9188, #10967, #583, #10757, #8861, #13988, #10860, #20687, #7327, #17503, #17606, #15855, #12302, #2460, #15968, #19030, #8976, #19363, #4228, #3904, #12421, #10645, #15756, #9735, #16395, #16287, #11290, #21565, #14745, #14851, #1008, #2896, #1121, #4454, #17937, #19902, #18157, #4776, #19471, #7757, #16605, #8190, #9834, #14641, #17838, #12867, #16182, #11507, #1231, #16498, #11408, #6422, #6096, #4342, #7974, #1443, #19586, #11083, #9517, #9630, #7864, #18040, #21451, #21239, #14964, #19789, #18250, #3109, #5979, #12750, #1333, #14523, #2684, #2782, #11185, #9414, #13192, #21345, #6203, #12974, #6308, #4663, #19682 ),
 .UNSPECIFIED., .F., .F.,
 ( 4, 3, 3, 3, 3, 3, 3, 3, 3, 3, 3, 3, 3, 3, 3, 3, 3, 3, 3, 3, 3, 3, 3, 3, 3, 3, 3, 3, 3, 3, 3, 3, 3, 3, 3, 3, 3, 3, 3, 3, 3, 3, 3, 3, 3, 3, 3, 3, 3, 3, 3, 3, 3, 3, 3, 3, 3, 3, 3, 3, 3, 3, 3, 3, 3, 3, 3, 3, 3, 3, 4 ),
 ( 0.000000000000000000, 0.01785714285713937630, 0.03571428571428875154, 0.04500001460683692583, 0.05357142857142812437, 0.07142857142856749719, 0.08928571428570687696, 0.1071428571428962584, 0.1100000694613451485, 0.1249999999999956285, 0.1428571428570949986, 0.1607142857142943582, 0.1749999145184668869, 0.1785714285713937421, 0.1964285714285931295, 0.2142857142856925134, 0.2321428571428918730, 0.2400000499947346211, 0.2499999999999912570, 0.2678571428570906132, 0.2857142857142900283, 0.3035714285713893568, 0.3050000289315413227, 0.3214285714285887163, 0.3392857142856881558, 0.3571428571428875154, 0.3699998972919570916, 0.3749999999999868994, 0.3928571428570862833, 0.4107142857142856429, 0.4285714285713849714, 0.4350000984216157995, 0.4464285714285843865, 0.4642857142856838260, 0.4821428571428831300, 0.4999999999999825140, 0.5178571428570818425, 0.5357142857142811465, 0.5535714285713807525, 0.5649999146099302649, 0.5714285714285800566, 0.5892857142856793295, 0.6071428571428788556, 0.6249999999999781286, 0.6300001157399379714, 0.6428571428570775126, 0.6607142857142768166, 0.6785714285713763116, 0.6949999841006686552, 0.6964285714285757267, 0.7142857142856749997, 0.7321428571428744148, 0.7499999999999737987, 0.7599999630366554015, 0.7678571428570730717, 0.7857142857142723757, 0.8035714285713719818, 0.8214285714285712858, 0.8250000985136630716, 0.8392857142856706698, 0.8571428571428700849, 0.8749999999999693578, 0.8899999435708758622, 0.8928571428570687418, 0.9107142857142680459, 0.9285714285713676519, 0.9464285714285669560, 0.9549999984243136009, 0.9642857142856662289, 0.9821428571428657550, 0.9999999999999650280 ),
 .UNSPECIFIED. ) ;
#13262=ORIENTED_EDGE ( 'NONE', *, *, #6028, .T. ) ;
#13323=CARTESIAN_POINT ( 'NONE',  ( 21.21496537101402424, -3.671282913444335438, -15.02289707828213139 ) ) ;
#13330=DIRECTION ( 'NONE',  ( -0.3482992169606098365, 0.9330960544336215357, -0.08955115110948595747 ) ) ;
#13332=CARTESIAN_POINT ( 'NONE',  ( 11.62339053785985676, -3.109361707316991019, -16.93227153458428447 ) ) ;
#13341=ADVANCED_FACE ( 'NONE', ( #1708 ), #16611, .T. ) ;
#13342=CARTESIAN_POINT ( 'NONE',  ( 11.75011716698597297, -4.547989565168462534, -16.18272918671651084 ) ) ;
#13348=CARTESIAN_POINT ( 'NONE',  ( 12.14154796308823236, -4.523627393238572658, -16.83224736341038508 ) ) ;
#13387=EDGE_CURVE ( 'NONE', #20548, #20642, #20712, .T. ) ;
#13390=FACE_OUTER_BOUND ( 'NONE', #1596, .T. ) ;
#13418=CARTESIAN_POINT ( 'NONE',  ( 11.97174136233939556, 21.25996874134203551, -17.62449286037261942 ) ) ;
#13419=CARTESIAN_POINT ( 'NONE',  ( 11.74417331903472395, -6.219808599076323219, -16.98778208059958317 ) ) ;
#13424=EDGE_CURVE ( 'NONE', #11296, #5048, #14475, .T. ) ;
#13430=CARTESIAN_POINT ( 'NONE',  ( 19.95088882991241164, -1.593704252466229931, -15.47347923388221425 ) ) ;
#13442=CARTESIAN_POINT ( 'NONE',  ( 10.41504388964860084, -3.120051954850537435, -17.35142295629939824 ) ) ;
#13448=CARTESIAN_POINT ( 'NONE',  ( 11.87836337660393582, -3.107092027145145874, -16.83199469523789915 ) ) ;
#13449=DIRECTION ( 'NONE',  ( -0.1132953773954069598, 0.7241889112991808375, -0.6802312681817410667 ) ) ;
#13509=SURFACE_STYLE_USAGE ( .BOTH. , #3336 ) ;
#13524=DIRECTION ( 'NONE',  ( -0.9161599507719021540, -0.3242921320961419940, -0.2355537256384720723 ) ) ;
#13533=LINE ( 'NONE', #5115, #10603 ) ;
#13535=CARTESIAN_POINT ( 'NONE',  ( 12.57351160526011924, -7.145082314903915766, -16.82041929937520663 ) ) ;
#13541=FACE_OUTER_BOUND ( 'NONE', #19666, .T. ) ;
#13543=CARTESIAN_POINT ( 'NONE',  ( 11.58844351015046215, -3.109292849304047035, -16.76334073837951877 ) ) ;
#13554=EDGE_CURVE ( 'NONE', #8439, #14268, #15210, .T. ) ;
#13559=CARTESIAN_POINT ( 'NONE',  ( 13.60955983258148727, -6.467614470005191407, -16.57130822712815998 ) ) ;
#13597=CARTESIAN_POINT ( 'NONE',  ( 19.30248346126309400, -5.034641893688545977, -14.21054282797976498 ) ) ;
#13598=ORIENTED_EDGE ( 'NONE', *, *, #7876, .T. ) ;
#13642=CARTESIAN_POINT ( 'NONE',  ( 20.24471977733230332, -1.311003557817993492, -14.75211372363476414 ) ) ;
#13646=CARTESIAN_POINT ( 'NONE',  ( 13.96963285379384878, -8.018802334511677898, -16.52276729540345457 ) ) ;
#13652=CARTESIAN_POINT ( 'NONE',  ( 17.21369304301024172, -7.336514211874763269, -15.87346308029872333 ) ) ;
#13654=VERTEX_POINT ( 'NONE', #604 ) ;
#13661=CARTESIAN_POINT ( 'NONE',  ( 17.36102099471316507, 2.301167714194472413, -15.54280354277228682 ) ) ;
#13669=CARTESIAN_POINT ( 'NONE',  ( 11.88276372161184113, -2.817112673463340933, -16.81723252566703053 ) ) ;
#13701=CARTESIAN_POINT ( 'NONE',  ( 15.97178949557365790, -7.235176167653088797, -14.86884501417147320 ) ) ;
#13709=EDGE_CURVE ( 'NONE', #12389, #736, #11104, .T. ) ;
#13756=CARTESIAN_POINT ( 'NONE',  ( 12.80420541122094846, -7.335296459352831810, -16.77213161543806308 ) ) ;
#13764=CARTESIAN_POINT ( 'NONE',  ( 11.76154713882772995, -4.503972587472946820, -15.73284477506779133 ) ) ;
#13766=DIRECTION ( 'NONE',  ( -0.3482992169606098365, 0.9330960544336215357, -0.08955115110948595747 ) ) ;
#13768=SHAPE_DEFINITION_REPRESENTATION ( #12499, #11147 ) ;
#13778=CARTESIAN_POINT ( 'NONE',  ( 18.19593279813170028, 0.2866705963667399715, -14.77465059166826578 ) ) ;
#13796=B_SPLINE_CURVE_WITH_KNOTS ( 'NONE', 3,
 ( #12606, #12393, #769, #20546, #8834 ),
 .UNSPECIFIED., .F., .F.,
 ( 4, 1, 4 ),
 ( 0.5007142149769521211, 0.7499992869954825725, 1.000000000000000000 ),
 .UNSPECIFIED. ) ;
#13812=CARTESIAN_POINT ( 'NONE',  ( 16.21443133523606406, -7.210654292967314305, -14.81810956799547974 ) ) ;
#13873=CARTESIAN_POINT ( 'NONE',  ( 17.67562427043129247, -8.149893664446995700, -15.71149448160998752 ) ) ;
#13905=CARTESIAN_POINT ( 'NONE',  ( 13.53491954000547537, 0.3256306608586702067, -16.21769529983032143 ) ) ;
#13907=VERTEX_POINT ( 'NONE', #3571 ) ;
#13918=ORIENTED_EDGE ( 'NONE', *, *, #13709, .F. ) ;
#13934=CARTESIAN_POINT ( 'NONE',  ( 17.80829803891473873, -6.635392327357950037, -14.48986153923296172 ) ) ;
#13940=CARTESIAN_POINT ( 'NONE',  ( 11.26949333533593922, -4.616615725918594038, -15.82154907933577448 ) ) ;
#13943=CARTESIAN_POINT ( 'NONE',  ( 17.90945013363836580, -8.300072463023354885, -14.29531981980184163 ) ) ;
#13949=CIRCLE ( 'NONE', #12164, 0.5953125000000005773 ) ;
#13961=( NAMED_UNIT ( * ) SI_UNIT ( $, .STERADIAN. ) SOLID_ANGLE_UNIT ( ) );
#13968=CIRCLE ( 'NONE', #15384, 0.5953125000000004663 ) ;
#13988=CARTESIAN_POINT ( 'NONE',  ( 19.93283111454340784, 0.1696482471589960683, -14.27155714560671207 ) ) ;
#13995=CARTESIAN_POINT ( 'NONE',  ( 11.63830738372303486, -3.658157632752987443, -15.74169750891422837 ) ) ;
#14002=CARTESIAN_POINT ( 'NONE',  ( 10.67348499102866555, -4.915146421765576257, -16.12107055749564921 ) ) ;
#14011=DIRECTION ( 'NONE',  ( -0.9037041334408598692, -0.3596272420165190220, -0.2323512126103423059 ) ) ;
#14022=CARTESIAN_POINT ( 'NONE',  ( 0.000000000000000000, 0.000000000000000000, 0.000000000000000000 ) ) ;
#14027=CARTESIAN_POINT ( 'NONE',  ( 20.37781590211399063, -3.328472077181156230, -15.39191602420292604 ) ) ;
#14037=CARTESIAN_POINT ( 'NONE',  ( 21.05604118250877477, -1.172420585967219653, -15.20663495340546412 ) ) ;
#14039=DIRECTION ( 'NONE',  ( -0.3140771401027085408, 0.9459569826691583971, -0.08075231887918271623 ) ) ;
#14047=CARTESIAN_POINT ( 'NONE',  ( 10.64919035412082238, -4.868472515922345423, -15.50245527337344420 ) ) ;
#14057=DIRECTION ( 'NONE',  ( -0.1132953773954069460, 0.7241889112991807265, -0.6802312681817409556 ) ) ;
#14065=ORIENTED_EDGE ( 'NONE', *, *, #19628, .T. ) ;
#14090=CARTESIAN_POINT ( 'NONE',  ( 17.29160225217250968, 2.068662977665156166, -15.07501658227938890 ) ) ;
#14102=ORIENTED_EDGE ( 'NONE', *, *, #19628, .F. ) ;
#14107=CARTESIAN_POINT ( 'NONE',  ( 17.31620997348098356, 2.440699290912120123, -15.21585355587603416 ) ) ;
#14115=CARTESIAN_POINT ( 'NONE',  ( 19.65947855433865143, -1.905983633164971769, -14.27020732896038346 ) ) ;
#14135=CARTESIAN_POINT ( 'NONE',  ( 19.39017462591846197, 0.4351151282638252571, -14.99845457969487583 ) ) ;
#14137=CARTESIAN_POINT ( 'NONE',  ( 12.51650226353079276, -6.117377381860210406, -15.54956597296763832 ) ) ;
#14149=CARTESIAN_POINT ( 'NONE',  ( 11.47063021243275394, -6.402320148554772494, -17.10925296469930146 ) ) ;
#14174=CARTESIAN_POINT ( 'NONE',  ( 11.83349417906578260, -4.444366718845225606, -15.99739072961142305 ) ) ;
#14203=CARTESIAN_POINT ( 'NONE',  ( 17.39128954282556450, 2.036810952640657479, -15.04541658584163777 ) ) ;
#14230=CARTESIAN_POINT ( 'NONE',  ( 12.54743718934339647, -0.7300314971274215470, -16.54148741527033906 ) ) ;
#14231=CARTESIAN_POINT ( 'NONE',  ( 13.28268573882264469, 19.39178765922512326, -19.83174211820151100 ) ) ;
#14235=CIRCLE ( 'NONE', #11398, 0.5953125000000005773 ) ;
#14247=CARTESIAN_POINT ( 'NONE',  ( 19.36302365051818342, 0.2638603526202955019, -15.04631431230876615 ) ) ;
#14249=CARTESIAN_POINT ( 'NONE',  ( 14.86522180462012876, -7.415116976227209555, -15.24400705011625767 ) ) ;
#14268=VERTEX_POINT ( 'NONE', #6835 ) ;
#14311=DIRECTION ( 'NONE',  ( -0.2490110332224889089, -7.284927983104707832E-16, 0.9685006480810781637 ) ) ;
#14312=CARTESIAN_POINT ( 'NONE',  ( 11.30450557499492348, -0.5489953149440882640, -16.88206917429806353 ) ) ;
#14330=DIRECTION ( 'NONE',  ( -0.1132953773954069598, 0.7241889112991808375, -0.6802312681817410667 ) ) ;
#14344=DIRECTION ( 'NONE',  ( 0.2490110332224855227, 0.000000000000000000, -0.9685006480810791629 ) ) ;
#14351=CARTESIAN_POINT ( 'NONE',  ( 19.45436729525584951, -5.351618512891932689, -14.30490051005982011 ) ) ;
#14363=CARTESIAN_POINT ( 'NONE',  ( 10.47858167127056106, -3.825101884021728349, -15.95313145255061116 ) ) ;
#14412=CARTESIAN_POINT ( 'NONE',  ( 14.35329266030264961, 2.065734012470558767, -15.94383203165788210 ) ) ;
#14436=ADVANCED_FACE ( 'NONE', ( #17218 ), #17977, .T. ) ;
#14445=CARTESIAN_POINT ( 'NONE',  ( 13.92886986911328506, 2.297057816795145424, -15.92078612283740569 ) ) ;
#14455=CARTESIAN_POINT ( 'NONE',  ( 19.61166229506757475, -5.924300855026435109, -15.80696905612679792 ) ) ;
#14475=B_SPLINE_CURVE_WITH_KNOTS ( 'NONE', 3,
 ( #8670, #8447, #3485, #10221, #10553, #7012, #384, #2029, #12223, #1818 ),
 .UNSPECIFIED., .F., .F.,
 ( 4, 2, 2, 2, 4 ),
 ( 0.000000000000000000, 0.2500000000000017764, 0.5000000000000011102, 0.7500000000000005551, 1.000000000000000000 ),
 .UNSPECIFIED. ) ;
#14523=CARTESIAN_POINT ( 'NONE',  ( 12.07693058128559649, -6.954572128932724695, -15.70789055935204281 ) ) ;
#14524=VECTOR ( 'NONE', #1036, 1000.000000000000000 ) ;
#14542=AXIS2_PLACEMENT_3D ( 'NONE', #3162, #4726, #19733 ) ;
#14547=CARTESIAN_POINT ( 'NONE',  ( 20.78426922154476131, -5.262943049308428378, -15.07321085010084438 ) ) ;
#14557=CARTESIAN_POINT ( 'NONE',  ( 19.70749945469935227, -6.234009617392132441, -14.61948376456804688 ) ) ;
#14573=CARTESIAN_POINT ( 'NONE',  ( 20.03605712096321412, -6.234006942471316925, -15.89736554983887906 ) ) ;
#14581=CARTESIAN_POINT ( 'NONE',  ( 20.08848443642310144, -3.313481494631655089, -15.32311112960731414 ) ) ;
#14603=CARTESIAN_POINT ( 'NONE',  ( 12.91059077353605211, 21.25996874134203907, -21.27604296009081253 ) ) ;
#14641=CARTESIAN_POINT ( 'NONE',  ( 17.96565374528240611, -7.898429124978179061, -14.43068046346296640 ) ) ;
#14647=CARTESIAN_POINT ( 'NONE',  ( 20.92131311655350245, -1.145359114192535888, -15.19233952661473097 ) ) ;
#14676=CARTESIAN_POINT ( 'NONE',  ( 13.89514527990785808, 2.161161825133189218, -15.59098570533049788 ) ) ;
#14685=CARTESIAN_POINT ( 'NONE',  ( 17.53610697582018574, -7.943091012973795273, -16.41972336742454530 ) ) ;
#14702=CARTESIAN_POINT ( 'NONE',  ( 10.63776237795206825, -4.912495182802602223, -15.95233917191240458 ) ) ;
#14745=CARTESIAN_POINT ( 'NONE',  ( 20.42592314637030881, -5.381782642937507077, -13.93043304647089187 ) ) ;
#14769=CARTESIAN_POINT ( 'NONE',  ( 21.02192561536538307, -1.427578428074376848, -15.15544506753321663 ) ) ;
#14778=CARTESIAN_POINT ( 'NONE',  ( 11.91437785957834983, -6.551758114717628700, -15.05791989401956776 ) ) ;
#14794=CARTESIAN_POINT ( 'NONE',  ( 20.09810219785228824, -3.122651124923756072, -15.32960905372040017 ) ) ;
#14805=CARTESIAN_POINT ( 'NONE',  ( 14.15750100853548510, -8.464140165015777484, -16.43479104712926642 ) ) ;
#14851=CARTESIAN_POINT ( 'NONE',  ( 20.35416303201372301, -5.534383657676722024, -13.94270872964028563 ) ) ;
#14874=CARTESIAN_POINT ( 'NONE',  ( 21.24317407479450281, -2.610281063246285616, -15.05445591060229660 ) ) ;
#14884=CARTESIAN_POINT ( 'NONE',  ( 19.50372870060111552, -0.8007013868912387089, -15.11219580267691143 ) ) ;
#14886=DIRECTION ( 'NONE',  ( -0.1132953773954069460, 0.7241889112991807265, -0.6802312681817409556 ) ) ;
#14893=CARTESIAN_POINT ( 'NONE',  ( 19.71456874936146875, -0.4919948594096015815, -14.92276603756576492 ) ) ;
#14897=CARTESIAN_POINT ( 'NONE',  ( 20.50301314505018624, -0.3073934294499542919, -15.81860185314828016 ) ) ;
#14964=CARTESIAN_POINT ( 'NONE',  ( 13.67320413129362677, -8.014437261679972835, -15.36892139067619212 ) ) ;
#14990=CARTESIAN_POINT ( 'NONE',  ( 20.92131311655350245, -1.145359114192535888, -15.19233952661473097 ) ) ;
#15001=CARTESIAN_POINT ( 'NONE',  ( 12.32505589497316478, -0.5459407413539660858, -16.45354645552742667 ) ) ;
#15009=CARTESIAN_POINT ( 'NONE',  ( 14.32880508193474256, -8.336696740575057163, -16.92443569652990476 ) ) ;
#15015=CARTESIAN_POINT ( 'NONE',  ( 17.19146193903594977, -7.054867240447602050, -15.83036007852367533 ) ) ;
#15027=ORIENTED_EDGE ( 'NONE', *, *, #11149, .F. ) ;
#15069=( NAMED_UNIT ( * ) PLANE_ANGLE_UNIT ( ) SI_UNIT ( $, .RADIAN. ) );
#15091=FACE_OUTER_BOUND ( 'NONE', #7373, .T. ) ;
#15092=CARTESIAN_POINT ( 'NONE',  ( 19.13395524456137053, -7.364572356485500570, -15.39828872268818927 ) ) ;
#15096=CARTESIAN_POINT ( 'NONE',  ( 21.05324281572633538, -1.171894783154180164, -15.19005319227003525 ) ) ;
#15102=CARTESIAN_POINT ( 'NONE',  ( 11.03537156866804025, -4.708219523321687916, -15.20365171484573708 ) ) ;
#15109=CARTESIAN_POINT ( 'NONE',  ( 21.08655736082664944, -1.169157187581218338, -15.28996091734704699 ) ) ;
#15118=CARTESIAN_POINT ( 'NONE',  ( 13.05392461046280417, -5.983512873707068636, -16.67921711117497097 ) ) ;
#15160=DIRECTION ( 'NONE',  ( -0.4128958666089267981, 0.5884034904305870395, 0.6951966166390379787 ) ) ;
#15170=ORIENTED_EDGE ( 'NONE', *, *, #18053, .T. ) ;
#15189=CARTESIAN_POINT ( 'NONE',  ( 19.99297611413309639, -0.4553737095896724374, -14.82343000113548648 ) ) ;
#15194=CARTESIAN_POINT ( 'NONE',  ( 12.35968435821843947, -6.936577703317105659, -16.86437037943348116 ) ) ;
#15202=CARTESIAN_POINT ( 'NONE',  ( 11.60004900376628711, -3.656864654387723679, -15.55631684518033886 ) ) ;
#15207=CARTESIAN_POINT ( 'NONE',  ( 13.62051399351888747, 17.23237496650334677, -17.80340391586448234 ) ) ;
#15210=CIRCLE ( 'NONE', #12018, 0.5953125000000004663 ) ;
#15218=CARTESIAN_POINT ( 'NONE',  ( 16.12778039609075265, -7.242576738085929833, -16.05200023831469025 ) ) ;
#15259=CARTESIAN_POINT ( 'NONE',  ( 13.04319607734463382, -6.245671925844710870, -15.47036368354625147 ) ) ;
#15308=CARTESIAN_POINT ( 'NONE',  ( 19.77720994532765530, -0.02498380418638844122, -14.87308496498962818 ) ) ;
#15311=CARTESIAN_POINT ( 'NONE',  ( 14.65205695078418380, -8.252331693867256845, -16.37421283785102233 ) ) ;
#15329=CARTESIAN_POINT ( 'NONE',  ( 11.68026082588236747, -6.323616958189365533, -17.48499852013087974 ) ) ;
#15373=CARTESIAN_POINT ( 'NONE',  ( 12.11768468619488637, -5.101415283429129310, -15.63842114478006629 ) ) ;
#15384=AXIS2_PLACEMENT_3D ( 'NONE', #3102, #6301, #13075 ) ;
#15421=CARTESIAN_POINT ( 'NONE',  ( 10.96829523475326695, -1.381748506594268733, -17.00159016424930414 ) ) ;
#15442=CARTESIAN_POINT ( 'NONE',  ( 13.34198401680142076, 0.1820865615191624709, -16.27895105414784638 ) ) ;
#15477=CARTESIAN_POINT ( 'NONE',  ( 15.48598371012319497, -7.240509137277070906, -14.97045021982148683 ) ) ;
#15508=ORIENTED_EDGE ( 'NONE', *, *, #13387, .T. ) ;
#15523=CARTESIAN_POINT ( 'NONE',  ( 19.76187703821956987, 0.0006356308824410450246, -14.87669286379018807 ) ) ;
#15527=CARTESIAN_POINT ( 'NONE',  ( 16.70007911672089662, -8.387532456226729494, -15.92482817259669581 ) ) ;
#15551=CARTESIAN_POINT ( 'NONE',  ( 12.83914629888907655, -0.3229198055095354736, -16.44254515780370696 ) ) ;
#15576=DIRECTION ( 'NONE',  ( -0.3482992169606098365, 0.9330960544336215357, -0.08955115110948595747 ) ) ;
#15579=CARTESIAN_POINT ( 'NONE',  ( 17.21645753443902649, -6.938450633991601002, -14.61028308222959637 ) ) ;
#15588=CARTESIAN_POINT ( 'NONE',  ( 10.65449937457216656, -4.912466459170417465, -16.01747763323893281 ) ) ;
#15589=ORIENTED_EDGE ( 'NONE', *, *, #1404, .F. ) ;
#15599=AXIS2_PLACEMENT_3D ( 'NONE', #7470, #17642, #14344 ) ;
#15641=CARTESIAN_POINT ( 'NONE',  ( 19.76338907927813437, -0.001881842415276016372, -14.87633619820457653 ) ) ;
#15645=CARTESIAN_POINT ( 'NONE',  ( 18.02971726292177124, 1.782683163403355309, -14.85524908451608006 ) ) ;
#15661=CARTESIAN_POINT ( 'NONE',  ( 11.66121486338230895, -6.991816407965024460, -15.94738478811983562 ) ) ;
#15670=CARTESIAN_POINT ( 'NONE',  ( 19.49661015955114607, -1.441193557778313483, -14.33538266661406979 ) ) ;
#15688=CARTESIAN_POINT ( 'NONE',  ( 11.74480790566189015, -4.503994935255103194, -15.66770688877914353 ) ) ;
#15701=CARTESIAN_POINT ( 'NONE',  ( 19.75795317206712198, -3.625818983740633605, -14.16333780485109273 ) ) ;
#15709=CARTESIAN_POINT ( 'NONE',  ( 19.84261803441996719, 0.4717451776687191511, -13.82102401822954718 ) ) ;
#15734=ORIENTED_EDGE ( 'NONE', *, *, #21383, .T. ) ;
#15755=DIRECTION ( 'NONE',  ( -0.3482992169606098365, 0.9330960544336215357, -0.08955115110948595747 ) ) ;
#15756=CARTESIAN_POINT ( 'NONE',  ( 20.91780793311170328, -3.648416207543188960, -13.87012058890019972 ) ) ;
#15762=CARTESIAN_POINT ( 'NONE',  ( 16.97011862608863098, 1.212343544023858355, -15.21366445222733077 ) ) ;
#15770=CARTESIAN_POINT ( 'NONE',  ( 20.34298345951636122, -6.628736041427409909, -15.10255183750635766 ) ) ;
#15778=CARTESIAN_POINT ( 'NONE',  ( 17.58887540853269371, 0.6711474593645572195, -14.96568140522104606 ) ) ;
#15791=CARTESIAN_POINT ( 'NONE',  ( 19.41351574269321389, 0.4248733107149043620, -14.98634048918820483 ) ) ;
#15792=ADVANCED_FACE ( 'NONE', ( #9376 ), #10033, .T. ) ;
#15794=CARTESIAN_POINT ( 'NONE',  ( 14.56131799329373600, -7.268434166347159220, -16.34826698112718901 ) ) ;
#15812=CARTESIAN_POINT ( 'NONE',  ( 10.83746537706882229, -3.114666494210958980, -16.41844068122003009 ) ) ;
#15831=ORIENTED_EDGE ( 'NONE', *, *, #4511, .T. ) ;
#15855=CARTESIAN_POINT ( 'NONE',  ( 20.67432262747533045, -1.268898791072118559, -14.02093111710477658 ) ) ;
#15882=CARTESIAN_POINT ( 'NONE',  ( 12.69615196668531709, -0.5037659573396899848, -16.49031973222839298 ) ) ;
#15905=CARTESIAN_POINT ( 'NONE',  ( 11.65751173500739846, -3.109302012046705421, -17.03197226462303249 ) ) ;
#15936=CARTESIAN_POINT ( 'NONE',  ( 20.09790673380831905, -2.779220565229514772, -15.34579478154137711 ) ) ;
#15939=CARTESIAN_POINT ( 'NONE',  ( 10.86025044861609601, -4.788864733524861528, -16.24762125301678850 ) ) ;
#15968=CARTESIAN_POINT ( 'NONE',  ( 20.88674645337222202, -2.120330402937725012, -13.93411895024804359 ) ) ;
#15994=MECHANICAL_DESIGN_GEOMETRIC_PRESENTATION_REPRESENTATION('',(#1491),#8887);
#16016=CARTESIAN_POINT ( 'NONE',  ( 16.94878383384984488, 1.210823707880592348, -15.13240640632768041 ) ) ;
#16028=EDGE_CURVE ( 'NONE', #11912, #736, #4513, .T. ) ;
#16059=EDGE_LOOP ( 'NONE', ( #17074, #1912, #814, #5225 ) ) ;
#16093=CARTESIAN_POINT ( 'NONE',  ( 11.37333528896229851, 0.1854951822871341027, -16.98463289171863977 ) ) ;
#16114=CARTESIAN_POINT ( 'NONE',  ( 19.67909734877197891, 0.1298811790940870847, -14.89708569419555317 ) ) ;
#16117=CARTESIAN_POINT ( 'NONE',  ( 12.56520165224167584, -6.111738713647066668, -15.71496090202399110 ) ) ;
#16127=ORIENTED_EDGE ( 'NONE', *, *, #11149, .T. ) ;
#16144=DIRECTION ( 'NONE',  ( 0.2490110332224869105, 8.271275069592406292E-16, -0.9685006480810787188 ) ) ;
#16182=CARTESIAN_POINT ( 'NONE',  ( 17.80487650496869279, -7.974366391153033362, -14.46540208612562317 ) ) ;
#16217=CARTESIAN_POINT ( 'NONE',  ( 10.49358939520456779, -3.807072909132312777, -15.50232714196991779 ) ) ;
#16225=CARTESIAN_POINT ( 'NONE',  ( 19.76774214424137099, -0.5915200861490187423, -14.90326874178355254 ) ) ;
#16226=CARTESIAN_POINT ( 'NONE',  ( 20.16764906325613893, -0.5540476120351953693, -16.10433982750742743 ) ) ;
#16234=PLANE ( 'NONE',  #13001 ) ;
#16239=CARTESIAN_POINT ( 'NONE',  ( 13.95773855287893461, 2.289327961384433063, -16.02183746796031372 ) ) ;
#16271=ORIENTED_EDGE ( 'NONE', *, *, #13709, .T. ) ;
#16287=CARTESIAN_POINT ( 'NONE',  ( 20.74198381141644631, -4.535585304848481769, -13.88224875571499162 ) ) ;
#16314=CARTESIAN_POINT ( 'NONE',  ( 21.15636133095030758, -2.013917305199845131, -15.09882835708281235 ) ) ;
#16322=CARTESIAN_POINT ( 'NONE',  ( 20.27068864692651573, -0.3073929331726920067, -14.91500286423835675 ) ) ;
#16330=CARTESIAN_POINT ( 'NONE',  ( 19.88373355471720316, -0.8065084006328289146, -14.86228188206940892 ) ) ;
#16332=CARTESIAN_POINT ( 'NONE',  ( 17.10804421600703051, 1.342424645466655964, -15.60784635835710255 ) ) ;
#16334=B_SPLINE_CURVE_WITH_KNOTS ( 'NONE', 3,
 ( #19113, #6251, #19224, #1177, #19627, #15936, #1059, #14794, #7805, #14581, #11232, #6150, #12918, #13025, #18207, #19846, #5627, #17981, #7918, #21398, #4603, #18096, #2955, #9681, #21505, #9885, #5137, #19955, #16654, #8125, #3597, #4827, #3279, #8446, #10011, #15015, #1497, #8345, #11888, #5235, #3157, #15218, #20371, #6689, #18728, #16765, #11562, #21732, #1604, #18299, #1817, #21621, #11784, #8242, #18616, #13559, #163, #4921, #15118, #16550, #6481, #18404, #5033, #1707, #13245, #6586, #10220, #20265, #13348, #21834, #3483, #16861, #18517, #8559, #6908, #13448, #20052, #11668, #13669, #3383, #20158, #10114, #47, #6801, #12325, #5803, #17420, #14230, #8770, #7135, #2374, #15882, #15551, #1925, #7456, #15442, #13905, #5687, #19052, #270, #17186, #20601, #603, #12559, #707, #20947, #19282, #18840, #8669, #10672, #10339, #12448, #4036, #2145, #12115, #5459, #2261, #9001, #3707, #17081, #15778, #7348, #10449, #13778, #9102, #20482, #12222, #2028, #18943, #10551, #5354, #19173, #3815, #10780, #17297, #15670, #8889, #14115, #20818, #17527, #3193, #8274, #10145, #5167, #196, #5492, #5267, #15701, #11820, #7278, #3413, #6938, #2062, #13597, #8595, #6837, #86, #416, #7046, #16891, #11918, #20632, #7170, #17220, #20298, #13934, #18549, #20518, #20199, #3850, #15579, #1741, #10478, #10372, #5386, #13812, #13701, #17118, #15477, #8480, #8698, #529, #20401, #12149, #5069, #18874, #2181, #10588, #10253, #8923, #12028, #1960, #15259, #3517, #303, #18647, #17000, #17333, #12252, #1854, #18761, #15373, #3631, #3743, #8803 ),
 .UNSPECIFIED., .F., .F.,
 ( 4, 3, 3, 3, 3, 3, 3, 3, 3, 3, 3, 3, 3, 3, 3, 3, 3, 3, 3, 3, 3, 3, 3, 3, 3, 3, 3, 3, 3, 3, 3, 3, 3, 3, 3, 3, 3, 3, 3, 3, 3, 3, 3, 3, 3, 3, 3, 3, 3, 3, 3, 3, 3, 3, 3, 3, 3, 3, 3, 3, 3, 3, 3, 3, 3, 3, 3, 3, 4 ),
 ( 3.118384633268010597E-11, 0.01886792455889550052, 0.03773584908660710530, 0.04500012977624090471, 0.05660377361432869514, 0.07547169814204039706, 0.09433962266975200184, 0.1099999085797309928, 0.1132075471974540032, 0.1320754717251650112, 0.1509433962528770046, 0.1698113207805879987, 0.1750001347259370066, 0.1886792453082999921, 0.2075471698360119854, 0.2264150943637230073, 0.2399998702385330029, 0.2452830188914350007, 0.2641509434191470218, 0.2830188679468579882, 0.3018867924745700093, 0.3050000920636670165, 0.3207547170022810312, 0.3396226415299929968, 0.3584905660577050179, 0.3699999077873000197, 0.3773584905854159843, 0.3962264151131280054, 0.4150943396408399710, 0.4339622641685509929, 0.4350000229552469788, 0.4528301886962630141, 0.4716981132239739805, 0.4905660377516860016, 0.5000000065312421027, 0.5094339622794979983, 0.5283018868072090202, 0.5471698113349209303, 0.5649999901081249609, 0.5660377358626329514, 0.5849056603903439733, 0.6037735849180559944, 0.6226415094457670163, 0.6300001052753160247, 0.6415094339734789264, 0.6603773585011909475, 0.6792452830289019694, 0.6949999209998329874, 0.6981132075566139905, 0.7169811320843260116, 0.7358490566120369225, 0.7547169811397489436, 0.7600001428246599966, 0.7735849056674599655, 0.7924528301951719866, 0.8113207547228840077, 0.8249998783372239908, 0.8301886792505950297, 0.8490566037783069397, 0.8679245283060189609, 0.8867924528337299828, 0.8900001044837360098, 0.9056603773614420039, 0.9245283018891530258, 0.9433962264168649359, 0.9549998832863340059, 0.9622641509445769570, 0.9811320754722879789, 1.000000000000000000 ),
 .UNSPECIFIED. ) ;
#16336=EDGE_CURVE ( 'NONE', #20642, #10436, #3692, .T. ) ;
#16395=CARTESIAN_POINT ( 'NONE',  ( 20.82425928449433528, -4.245348575377335898, -13.87212089903126078 ) ) ;
#16423=DIRECTION ( 'NONE',  ( -0.4128958666089269647, 0.5884034904305883718, 0.6951966166390366464 ) ) ;
#16433=CARTESIAN_POINT ( 'NONE',  ( 19.40057331552889153, -5.839280184494942461, -15.41429742563731864 ) ) ;
#16441=CARTESIAN_POINT ( 'NONE',  ( 19.55894973361720091, -0.1923335449227899507, -14.98190768515691751 ) ) ;
#16443=CARTESIAN_POINT ( 'NONE',  ( 20.83211096346473568, -2.693633402772701579, -14.60905691900277148 ) ) ;
#16455=CARTESIAN_POINT ( 'NONE',  ( 11.62409918280433985, -6.986177739752845284, -15.77901157387964126 ) ) ;
#16498=CARTESIAN_POINT ( 'NONE',  ( 17.13928781705268989, -8.220053430339435252, -14.61006923465378904 ) ) ;
#16526=CARTESIAN_POINT ( 'NONE',  ( 20.50050043015025025, -0.2396794266589334643, -15.37230335780461310 ) ) ;
#16534=CARTESIAN_POINT ( 'NONE',  ( 19.38529025477529899, -5.351634827297560904, -14.03627082355416178 ) ) ;
#16535=LINE ( 'NONE', #1366, #18744 ) ;
#16541=CARTESIAN_POINT ( 'NONE',  ( 19.40504022072852663, 0.1453320723159260697, -15.03681954599216652 ) ) ;
#16542=AXIS2_PLACEMENT_3D ( 'NONE', #8518, #6873, #16823 ) ;
#16543=CARTESIAN_POINT ( 'NONE',  ( 17.61528648211390902, -7.258561849689513679, -14.99581366938190818 ) ) ;
#16550=CARTESIAN_POINT ( 'NONE',  ( 12.88764127389737446, -5.800509336186265408, -16.71032010666468537 ) ) ;
#16605=CARTESIAN_POINT ( 'NONE',  ( 18.72668781722862263, -7.437140393198111710, -14.26808916428128349 ) ) ;
#16611=TOROIDAL_SURFACE ( 'NONE', #3905, 3.174999999999999822, 0.5953125000000000222 ) ;
#16636=CARTESIAN_POINT ( 'NONE',  ( 20.35960306314353474, -3.328948665870211432, -15.28812545466150219 ) ) ;
#16640=EDGE_LOOP ( 'NONE', ( #5415, #12246 ) ) ;
#16644=CARTESIAN_POINT ( 'NONE',  ( 21.56000048501562816, -3.394315525992640303, -15.42643609242808367 ) ) ;
#16654=CARTESIAN_POINT ( 'NONE',  ( 18.39685687182289797, -6.445242814774206686, -15.58509951939779370 ) ) ;
#16740=CARTESIAN_POINT ( 'NONE',  ( 11.94887888776901441, -6.501231973260999553, -16.94794046497096573 ) ) ;
#16750=CARTESIAN_POINT ( 'NONE',  ( 16.92054404696516912, 1.202889707813861619, -15.03119329449350339 ) ) ;
#16765=CARTESIAN_POINT ( 'NONE',  ( 15.16174527195880017, -7.152427045711343467, -16.25377686098167374 ) ) ;
#16823=DIRECTION ( 'NONE',  ( 0.3697464814795228816, -0.9291326812858931028, 0.000000000000000000 ) ) ;
#16832=CARTESIAN_POINT ( 'NONE',  ( 20.24085330020690066, -1.338735640124543602, -14.75261804466661353 ) ) ;
#16835=CARTESIAN_POINT ( 'NONE',  ( 18.11329111247768253, -7.967937188882820543, -15.61660755156637315 ) ) ;
#16847=CARTESIAN_POINT ( 'NONE',  ( 14.79613284372093318, -7.415112926742073896, -14.97538028618549610 ) ) ;
#16861=CARTESIAN_POINT ( 'NONE',  ( 11.94302826524597805, -3.805938227851652478, -16.84833834122463614 ) ) ;
#16891=CARTESIAN_POINT ( 'NONE',  ( 18.89948197725901124, -5.655894340861864933, -14.27920814860754817 ) ) ;
#16897=EDGE_LOOP ( 'NONE', ( #963, #4739, #13262, #18359, #7896 ) ) ;
#16933=CARTESIAN_POINT ( 'NONE',  ( 19.74554184638576260, 0.02755205230605372105, -14.88057453995056889 ) ) ;
#16937=CARTESIAN_POINT ( 'NONE',  ( 11.77229620076644956, -6.258712276749109016, -16.98231560743968416 ) ) ;
#17000=CARTESIAN_POINT ( 'NONE',  ( 12.65199039493287358, -5.861692353372749409, -15.54496691525876528 ) ) ;
#17017=AXIS2_PLACEMENT_3D ( 'NONE', #11380, #5846, #12604 ) ;
#17053=CARTESIAN_POINT ( 'NONE',  ( 16.11221013415338632, -8.434765728320028799, -16.05392306811195269 ) ) ;
#17074=ORIENTED_EDGE ( 'NONE', *, *, #13424, .T. ) ;
#17081=CARTESIAN_POINT ( 'NONE',  ( 17.37611761637614194, 0.7803472578652853597, -15.03203363529809167 ) ) ;
#17118=CARTESIAN_POINT ( 'NONE',  ( 15.72888660284841755, -7.237842652465062088, -14.91964761699648889 ) ) ;
#17163=CARTESIAN_POINT ( 'NONE',  ( 20.16676785488811419, -0.9350613415272122086, -14.77802399055632776 ) ) ;
#17166=CARTESIAN_POINT ( 'NONE',  ( 19.36645978477608310, -7.176659453237705932, -15.34953550627761842 ) ) ;
#17172=CARTESIAN_POINT ( 'NONE',  ( 19.95643545564609056, -1.593178449655435092, -15.48935439063656538 ) ) ;
#17180=CARTESIAN_POINT ( 'NONE',  ( 20.48137360697176490, -5.937212919150582913, -14.37931843660670062 ) ) ;
#17186=CARTESIAN_POINT ( 'NONE',  ( 14.25471133999911011, 0.7535054429800847053, -15.99185436641439217 ) ) ;
#17197=CYLINDRICAL_SURFACE ( 'NONE', #1793, 0.5953124999999994671 ) ;
#17218=FACE_OUTER_BOUND ( 'NONE', #16897, .T. ) ;
#17220=CARTESIAN_POINT ( 'NONE',  ( 18.21294863246763640, -6.358645335814493649, -14.40912211738714888 ) ) ;
#17227=CARTESIAN_POINT ( 'NONE',  ( 17.24715906500612306, 2.440694956846978680, -14.94721736399773704 ) ) ;
#17231=APPLICATION_CONTEXT ( 'automotive_design' ) ;
#17270=CARTESIAN_POINT ( 'NONE',  ( 20.18678758757129543, -1.006362617683279836, -14.77198301169015693 ) ) ;
#17274=CARTESIAN_POINT ( 'NONE',  ( 16.07189111700614603, 2.286673086399800159, -15.43580752111316556 ) ) ;
#17282=CARTESIAN_POINT ( 'NONE',  ( 12.53323336751100392, -6.117360363457603256, -15.61470599677969595 ) ) ;
#17288=CARTESIAN_POINT ( 'NONE',  ( 14.61877701993662981, -8.672575780289569991, -15.30737042585371377 ) ) ;
#17297=CARTESIAN_POINT ( 'NONE',  ( 19.40549191052905798, -1.213055114509968613, -14.37046020240782518 ) ) ;
#17314=ORIENTED_EDGE ( 'NONE', *, *, #20823, .F. ) ;
#17333=CARTESIAN_POINT ( 'NONE',  ( 12.58984874085997419, -5.789910881123263131, -15.55645878085723233 ) ) ;
#17343=CARTESIAN_POINT ( 'NONE',  ( 10.34597555076318187, -3.120040139117916222, -17.08279145937373045 ) ) ;
#17350=ADVANCED_FACE ( 'NONE', ( #12136, #12801 ), #7909, .T. ) ;
#17364=CARTESIAN_POINT ( 'NONE',  ( 11.85370378511233191, -4.423560566297380703, -15.83226420197127204 ) ) ;
#17398=CARTESIAN_POINT ( 'NONE',  ( 15.49294960918546238, 2.279643855968550792, -15.60671101686425288 ) ) ;
#17407=CARTESIAN_POINT ( 'NONE',  ( 19.52837946232106248, -0.8676311488457835175, -15.63954645954029843 ) ) ;
#17420=CARTESIAN_POINT ( 'NONE',  ( 12.41531557771041783, -0.9351939426588545823, -16.58710729350898561 ) ) ;
#17437=CARTESIAN_POINT ( 'NONE',  ( 19.42680641351661919, 0.4165720343021085958, -14.98010323326712268 ) ) ;
#17440=CARTESIAN_POINT ( 'NONE',  ( 12.43890308457113747, -5.664764769703692693, -16.75625553099141385 ) ) ;
#17441=ORIENTED_EDGE ( 'NONE', *, *, #19305, .T. ) ;
#17457=CARTESIAN_POINT ( 'NONE',  ( 20.48685332741090903, -6.007402871720267434, -13.93096415391416976 ) ) ;
#17499=DIRECTION ( 'NONE',  ( -0.3482992169606098365, 0.9330960544336215357, -0.08955115110948595747 ) ) ;
#17503=CARTESIAN_POINT ( 'NONE',  ( 20.45273674534495711, -0.7129475169430978809, -14.09995496590185304 ) ) ;
#17517=CARTESIAN_POINT ( 'NONE',  ( 21.32189013745294659, -2.645762206214888224, -13.94514596636895298 ) ) ;
#17527=CARTESIAN_POINT ( 'NONE',  ( 19.75297330285050279, -2.349405567017404106, -14.22479102338560253 ) ) ;
#17543=ORIENTED_EDGE ( 'NONE', *, *, #1308, .F. ) ;
#17544=CARTESIAN_POINT ( 'NONE',  ( 19.33880417540428098, 0.3883429578762613854, -15.04034309088197574 ) ) ;
#17546=CARTESIAN_POINT ( 'NONE',  ( 19.41828633390691294, -5.355847088986745774, -14.13626125933856592 ) ) ;
#17595=CIRCLE ( 'NONE', #16542, 2.579687500000000355 ) ;
#17606=CARTESIAN_POINT ( 'NONE',  ( 20.56352968641046886, -0.9909231540084149081, -14.06044304150320556 ) ) ;
#17642=DIRECTION ( 'NONE',  ( -0.3482992169606098365, 0.9330960544336215357, -0.08955115110948595747 ) ) ;
#17644=DIRECTION ( 'NONE',  ( 1.000000000000000000, 0.000000000000000000, 0.000000000000000000 ) ) ;
#17652=CARTESIAN_POINT ( 'NONE',  ( 19.36991330292439173, 0.2418614478177981975, -15.04532736253224989 ) ) ;
#17653=CARTESIAN_POINT ( 'NONE',  ( 14.82073529532191714, -7.423173529680283877, -15.07752894836403890 ) ) ;
#17654=EDGE_LOOP ( 'NONE', ( #10884, #18306, #15027, #20822 ) ) ;
#17698=ORIENTED_EDGE ( 'NONE', *, *, #3696, .T. ) ;
#17720=CARTESIAN_POINT ( 'NONE',  ( 11.45318987056821136, -0.2908542355871540641, -16.83281496953432210 ) ) ;
#17745=COLOUR_RGB ( '', 0.66274510, 0.83137255, 0.94901961) ;
#17770=CARTESIAN_POINT ( 'NONE',  ( 14.64275916103558650, -7.397369947662747691, -16.84371501784351466 ) ) ;
#17838=CARTESIAN_POINT ( 'NONE',  ( 17.91249156466048831, -7.924689752748640181, -14.44214372066701735 ) ) ;
#17866=CARTESIAN_POINT ( 'NONE',  ( 21.03152454542845717, -2.656576306117378827, -13.39494047124001952 ) ) ;
#17874=CARTESIAN_POINT ( 'NONE',  ( 20.15758252994617550, -1.280876140752218895, -14.77588887141922847 ) ) ;
#17875=CARTESIAN_POINT ( 'NONE',  ( 14.37725694972261081, 1.099222879083521676, -15.91397516589488781 ) ) ;
#17887=CARTESIAN_POINT ( 'NONE',  ( 13.95408900351856119, 2.287844446565507450, -16.00547455423211574 ) ) ;
#17937=CARTESIAN_POINT ( 'NONE',  ( 19.97525939775061232, -6.161891578892464416, -14.01322510184426662 ) ) ;
#17969=CARTESIAN_POINT ( 'NONE',  ( 21.28779318124766107, -2.646397705288468405, -13.84543864803846880 ) ) ;
#17976=CARTESIAN_POINT ( 'NONE',  ( 19.50266732720887219, -0.07610042702671838966, -15.00324811268347602 ) ) ;
#17977=B_SPLINE_SURFACE_WITH_KNOTS ( 'NONE', 3, 3, ( 
 ( #7276, #14037, #20742, #2292, #20851, #7377, #14149, #3515, #5724, #194, #6936, #2813, #5692, #7679, #5809, #12665, #21156, #12783, #19506 ),
 ( #16526, #15096, #11538, #1160, #10486, #7899, #6132, #5500, #7285, #4482, #3858, #12371, #17969, #17457, #13011, #2070, #19715, #15588, #19098 ),
 ( #10596, #20755, #18985, #12262, #12903, #19512, #7178, #17343, #2300, #14445, #17227, #19615, #2191, #21276, #13943, #8932, #21384, #7388, #20640 ),
 ( #16322, #11218, #4380, #3967, #21162, #6017, #8811, #12789, #2711, #14676, #11114, #15709, #17866, #9445, #2819, #9554, #537, #14047, #16217 ),
 ( #1044, #7789, #5611, #14557, #10712, #9037, #638, #15812, #19939, #21487, #3043, #13229, #8007, #5016, #18079, #21717, #14778, #15102, #1591 ),
 ( #14884, #11545, #4587, #11329, #3259, #2939, #21603, #18283, #11653, #3144, #30, #4903, #10100, #9868, #6570, #6343, #11771, #9995, #8333 ),
 ( #6669, #1264, #6465, #1687, #18387, #4812, #21816, #13543, #15001, #6782, #16750, #8426, #9768, #16534, #18496, #16847, #1364, #9664, #15202 ),
 ( #8107, #13430, #16636, #16433, #11445, #13117, #3368, #13332, #20141, #19830, #4705, #18190, #1479, #20034, #8226, #484, #17282, #13764, #5332 ),
 ( #17407, #17172, #5553, #3469, #13652, #3689, #2012, #6891, #10203, #12310, #15762, #8653, #20353, #5222, #20464, #5124, #7237, #18602, #13995 ) ),
 .UNSPECIFIED., .F., .F., .F.,
 ( 4, 1, 1, 1, 1, 1, 4 ),
 ( 4, 1, 1, 1, 1, 1, 1, 1, 1, 1, 1, 1, 1, 1, 1, 1, 4 ),
 ( 0.4864838642302999894, 0.5000000000000000000, 0.6250000000000000000, 0.7500000000000000000, 0.8750000000000000000, 1.000000000000000000, 1.013516135769999993 ),
 ( -0.02000001207767999889, 0.04500002717478000097, 0.1100000664272000050, 0.1750001056797000076, 0.2400001449321000069, 0.3050001841846000095, 0.3700002234370000087, 0.4350002626895000390, 0.5000003019419000383, 0.5650003411944000131, 0.6300003804468999880, 0.6950004196992999317, 0.7600004589518000175, 0.8250004982041999613, 0.8900005374567000471, 0.9550005767090999909, 1.020000615962000090 ),
 .UNSPECIFIED. ) ;
#17981=CARTESIAN_POINT ( 'NONE',  ( 19.65195596176846848, -4.944832552674430559, -15.35560206351170898 ) ) ;
#18040=CARTESIAN_POINT ( 'NONE',  ( 14.51424632332418163, -8.292823964279493865, -15.18575921541595974 ) ) ;
#18053=EDGE_CURVE ( 'NONE', #13084, #13225, #5280, .T. ) ;
#18079=CARTESIAN_POINT ( 'NONE',  ( 17.52900673049509805, -7.713162168938938024, -13.85515164265490462 ) ) ;
#18087=CARTESIAN_POINT ( 'NONE',  ( 19.83216830577377365, -0.7115147061423999775, -14.88007337591235846 ) ) ;
#18096=CARTESIAN_POINT ( 'NONE',  ( 19.18622267977934470, -5.669706517139640134, -15.43468797119958502 ) ) ;
#18118=DIRECTION ( 'NONE',  ( -0.3482992169606098365, 0.9330960544336215357, -0.08955115110948595747 ) ) ;
#18140=B_SPLINE_CURVE_WITH_KNOTS ( 'NONE', 3,
 ( #9050, #17364, #14174, #10728, #654, #7400, #2431, #15939, #767, #7518 ),
 .UNSPECIFIED., .F., .F.,
 ( 4, 2, 2, 2, 4 ),
 ( 0.000000000000000000, 0.2500000000000000000, 0.5000000000000000000, 0.7500000000000000000, 1.000000000000000000 ),
 .UNSPECIFIED. ) ;
#18157=CARTESIAN_POINT ( 'NONE',  ( 19.61169252880100089, -6.639328201340718216, -14.08464967305818938 ) ) ;
#18181=CARTESIAN_POINT ( 'NONE',  ( 19.76333778421562215, -6.796690732811715208, -15.26778210143417702 ) ) ;
#18184=FACE_OUTER_BOUND ( 'NONE', #4593, .T. ) ;
#18190=CARTESIAN_POINT ( 'NONE',  ( 19.12285863748637382, -0.2473773731819471633, -14.52246859281454761 ) ) ;
#18197=CARTESIAN_POINT ( 'NONE',  ( 19.43379288100138069, 0.07459186394039191148, -15.02802818531180584 ) ) ;
#18201=CARTESIAN_POINT ( 'NONE',  ( 12.54492807148089284, -6.210945379539458244, -16.05864477962155590 ) ) ;
#18207=CARTESIAN_POINT ( 'NONE',  ( 19.92484631573285370, -4.252746759165957791, -15.32038969226572256 ) ) ;
#18219=ORIENTED_EDGE ( 'NONE', *, *, #13554, .F. ) ;
#18250=CARTESIAN_POINT ( 'NONE',  ( 13.13857632649210672, -7.757696357571966850, -15.48432750494124832 ) ) ;
#18283=CARTESIAN_POINT ( 'NONE',  ( 11.36675820428501282, -3.110504336422511340, -16.48186686805254908 ) ) ;
#18293=CARTESIAN_POINT ( 'NONE',  ( 20.07739328931695511, -1.153533769354293748, -14.79997852497580979 ) ) ;
#18295=CARTESIAN_POINT ( 'NONE',  ( 14.34014943933268071, 1.694275420233978036, -16.63941580623522398 ) ) ;
#18299=CARTESIAN_POINT ( 'NONE',  ( 14.59124287633469308, -6.988731851215915114, -16.37203253287690785 ) ) ;
#18306=ORIENTED_EDGE ( 'NONE', *, *, #797, .T. ) ;
#18334=ORIENTED_EDGE ( 'NONE', *, *, #9671, .T. ) ;
#18359=ORIENTED_EDGE ( 'NONE', *, *, #3420, .T. ) ;
#18376=CARTESIAN_POINT ( 'NONE',  ( 13.04853822875846348, -7.504789825882131282, -16.72033722309888759 ) ) ;
#18386=DIRECTION ( 'NONE',  ( 0.2490110332224855227, 0.000000000000000000, -0.9685006480810791629 ) ) ;
#18387=CARTESIAN_POINT ( 'NONE',  ( 17.16396544380940270, -7.327104899143136230, -15.69103126553038408 ) ) ;
#18396=CARTESIAN_POINT ( 'NONE',  ( 14.91906957739207762, -7.556863888178527944, -15.56863359939283242 ) ) ;
#18404=CARTESIAN_POINT ( 'NONE',  ( 12.71419532639660588, -5.571168796945357826, -16.74134232755136864 ) ) ;
#18436=CIRCLE ( 'NONE', #19151, 0.5953125000000005773 ) ;
#18490=CARTESIAN_POINT ( 'NONE',  ( 13.81931296094454531, -7.948541684644407468, -16.55524147760729647 ) ) ;
#18496=CARTESIAN_POINT ( 'NONE',  ( 17.40805163412996492, -7.126251874856905921, -14.42423430082585156 ) ) ;
#18508=CARTESIAN_POINT ( 'NONE',  ( 20.53300515663952908, -0.2355993312742575563, -15.47241927149025109 ) ) ;
#18517=CARTESIAN_POINT ( 'NONE',  ( 11.91164091833190852, -3.559739266059170681, -16.84475823795191829 ) ) ;
#18549=CARTESIAN_POINT ( 'NONE',  ( 17.65755290411736311, -6.728872469205175122, -14.52017334799040782 ) ) ;
#18559=ORIENTED_EDGE ( 'NONE', *, *, #9773, .F. ) ;
#18561=EDGE_CURVE ( 'NONE', #11296, #19395, #13533, .T. ) ;
#18588=CARTESIAN_POINT ( 'NONE',  ( 20.23691056526638832, -1.234862104235166402, -14.75547226453677219 ) ) ;
#18591=CARTESIAN_POINT ( 'NONE',  ( 10.72696675674987254, -2.863640533428135626, -17.11876806796568573 ) ) ;
#18602=CARTESIAN_POINT ( 'NONE',  ( 11.76433965462081055, -4.504481791847095629, -15.74942804055007706 ) ) ;
#18610=CARTESIAN_POINT ( 'NONE',  ( 11.57003115466494769, 0.1030431252659232133, -17.27253179266325489 ) ) ;
#18616=CARTESIAN_POINT ( 'NONE',  ( 13.81552360302172922, -6.599745701269019271, -16.53000304243150964 ) ) ;
#18647=CARTESIAN_POINT ( 'NONE',  ( 12.71652186471789037, -5.931147806008448597, -15.53286060487739029 ) ) ;
#18701=CARTESIAN_POINT ( 'NONE',  ( 10.72385252731403860, -3.032576214141862625, -17.12574345756441119 ) ) ;
#18728=CARTESIAN_POINT ( 'NONE',  ( 15.39982685781387239, -7.202102660715429039, -16.20421384448473745 ) ) ;
#18744=VECTOR ( 'NONE', #14886, 1000.000000000000114 ) ;
#18761=CARTESIAN_POINT ( 'NONE',  ( 12.23724559180106297, -5.318041355315282992, -15.61933097726557662 ) ) ;
#18773=AXIS2_PLACEMENT_3D ( 'NONE', #13940, #10258, #2067 ) ;
#18814=CARTESIAN_POINT ( 'NONE',  ( 18.88804190845695530, -7.531632358019679785, -15.45048948743678352 ) ) ;
#18840=CARTESIAN_POINT ( 'NONE',  ( 15.27944507982620692, 1.059665764626953388, -15.67595978355573116 ) ) ;
#18865=VECTOR ( 'NONE', #14057, 1000.000000000000114 ) ;
#18874=CARTESIAN_POINT ( 'NONE',  ( 14.48894653437083058, -7.059436537805347633, -15.17821728035911910 ) ) ;
#18903=ORIENTED_EDGE ( 'NONE', *, *, #18561, .T. ) ;
#18918=CARTESIAN_POINT ( 'NONE',  ( 20.20352062662200154, -1.069946468824292563, -14.76680097212925347 ) ) ;
#18922=CARTESIAN_POINT ( 'NONE',  ( 16.64770984238460372, 2.218310395241972266, -15.26570684048795457 ) ) ;
#18943=CARTESIAN_POINT ( 'NONE',  ( 18.85280999513622646, -0.3457920826010936199, -14.56172347197127692 ) ) ;
#18969=CARTESIAN_POINT ( 'NONE',  ( 19.88300675555340291, -1.573955445284405785, -15.61985652438219496 ) ) ;
#18985=CARTESIAN_POINT ( 'NONE',  ( 21.54912629262006973, -3.402682142040095670, -14.80437132354864715 ) ) ;
#19026=CARTESIAN_POINT ( 'NONE',  ( 20.23139908883704763, -1.200391101382722203, -14.75749743533480007 ) ) ;
#19030=CARTESIAN_POINT ( 'NONE',  ( 20.92591353227786044, -2.395484007738812871, -13.91390478273180165 ) ) ;
#19052=CARTESIAN_POINT ( 'NONE',  ( 13.93302862726156199, 0.5950094174631964661, -16.09203730721210235 ) ) ;
#19073=CARTESIAN_POINT ( 'NONE',  ( 19.14286813974102586, -0.2525960963907294965, -14.62579786283977867 ) ) ;
#19098=CARTESIAN_POINT ( 'NONE',  ( 10.49532457957784359, -3.825071637629403387, -16.01826837021063099 ) ) ;
#19113=CARTESIAN_POINT ( 'NONE',  ( 19.84534036711146143, -1.573540299197002224, -15.46898262837090243 ) ) ;
#19149=CARTESIAN_POINT ( 'NONE',  ( 11.84053051238870147, 0.2936998923501951686, -16.70720445209922289 ) ) ;
#19151=AXIS2_PLACEMENT_3D ( 'NONE', #8106, #21815, #18386 ) ;
#19173=CARTESIAN_POINT ( 'NONE',  ( 19.08799226225449885, -0.6592077476704274464, -14.48249918540156855 ) ) ;
#19190=CARTESIAN_POINT ( 'NONE',  ( 19.36217743480797893, 0.4374727505662669436, -15.01545013472033396 ) ) ;
#19193=PRODUCT ( 'Handle Pawl Torsion Spring', 'Handle Pawl Torsion Spring', '', ( #20806 ) ) ;
#19194=CARTESIAN_POINT ( 'NONE',  ( 12.51121735021641612, -6.118460377156197616, -15.53362352737866736 ) ) ;
#19224=CARTESIAN_POINT ( 'NONE',  ( 19.99079755883271758, -2.044740353336991223, -15.40828390584228202 ) ) ;
#19259=CARTESIAN_POINT ( 'NONE',  ( 17.48992360529581092, 2.001781804147173549, -15.01608738236844687 ) ) ;
#19282=CARTESIAN_POINT ( 'NONE',  ( 15.04459320328107630, 1.018023609948645269, -15.74799260762002540 ) ) ;
#19300=CARTESIAN_POINT ( 'NONE',  ( 19.10310856060884532, -0.2463609076444987778, -14.44080317216485376 ) ) ;
#19305=EDGE_CURVE ( 'NONE', #5048, #11296, #18140, .T. ) ;
#19313=CARTESIAN_POINT ( 'NONE',  ( 14.57744845994609584, -8.664519226834075383, -15.14008038430411140 ) ) ;
#19363=CARTESIAN_POINT ( 'NONE',  ( 20.94506505885473757, -2.696405856112658928, -13.89795473303651008 ) ) ;
#19380=ORIENTED_EDGE ( 'NONE', *, *, #3696, .F. ) ;
#19395=VERTEX_POINT ( 'NONE', #9487 ) ;
#19403=ADVANCED_FACE ( 'NONE', ( #4633 ), #12800, .T. ) ;
#19404=CARTESIAN_POINT ( 'NONE',  ( 19.73605314530132304, -0.8007017946179174617, -16.01579480532253186 ) ) ;
#19417=CARTESIAN_POINT ( 'NONE',  ( 20.04694561498230598, 0.5575515236321860746, -14.19813339123195561 ) ) ;
#19429=CYLINDRICAL_SURFACE ( 'NONE', #778, 0.5953125000000005773 ) ;
#19471=CARTESIAN_POINT ( 'NONE',  ( 19.19346778367484774, -7.066212543700896020, -14.17012739972722279 ) ) ;
#19497=AXIS2_PLACEMENT_3D ( 'NONE', #3310, #11914, #20082 ) ;
#19506=CARTESIAN_POINT ( 'NONE',  ( 10.50091842137632270, -3.824863312786503045, -16.03413138725077403 ) ) ;
#19512=CARTESIAN_POINT ( 'NONE',  ( 14.13241029341496358, -8.473400452264066018, -16.35006988243831927 ) ) ;
#19524=CARTESIAN_POINT ( 'NONE',  ( 19.54280466309461062, -0.8724958927937114250, -15.72700954820671626 ) ) ;
#19540=CARTESIAN_POINT ( 'NONE',  ( 21.03094872803853121, -1.172420608524037178, -15.10904117410172276 ) ) ;
#19552=CARTESIAN_POINT ( 'NONE',  ( 14.93145837000203358, 15.36419388438619826, -20.01065317369261365 ) ) ;
#19586=CARTESIAN_POINT ( 'NONE',  ( 15.14187524152246844, -8.405880411091629867, -15.04820586386156478 ) ) ;
#19615=CARTESIAN_POINT ( 'NONE',  ( 20.03229091909386739, 0.5637714581750892240, -14.11072859660528955 ) ) ;
#19627=CARTESIAN_POINT ( 'NONE',  ( 20.07602185242275894, -2.531604885293976981, -15.36307167742676327 ) ) ;
#19628=EDGE_CURVE ( 'NONE', #8439, #9259, #6062, .T. ) ;
#19666=EDGE_LOOP ( 'NONE', ( #15589, #17441, #18903, #9737 ) ) ;
#19682=CARTESIAN_POINT ( 'NONE',  ( 10.72409186464205355, -4.809670885807086016, -15.96177715662992824 ) ) ;
#19715=CARTESIAN_POINT ( 'NONE',  ( 11.64082572770862889, -6.986155865975274715, -15.84415276987491339 ) ) ;
#19733=DIRECTION ( 'NONE',  ( -0.9161599507719021540, -0.3242921320961419940, -0.2355537256384720723 ) ) ;
#19737=CARTESIAN_POINT ( 'NONE',  ( 17.26663542346604174, 2.431245447269064108, -15.03338239065812232 ) ) ;
#19789=CARTESIAN_POINT ( 'NONE',  ( 13.40114476004444377, -7.897675722708163981, -15.42784453033882031 ) ) ;
#19814=CIRCLE ( 'NONE', #11008, 2.579687500000000355 ) ;
#19819=CARTESIAN_POINT ( 'NONE',  ( 21.10104941149074520, -1.718252868000626155, -15.12407559264656776 ) ) ;
#19830=CARTESIAN_POINT ( 'NONE',  ( 14.39401533775971131, 1.099227433804672138, -15.97910867269435720 ) ) ;
#19839=CARTESIAN_POINT ( 'NONE',  ( 14.53389803956520332, -7.867033344118881999, -17.07121685545881817 ) ) ;
#19846=CARTESIAN_POINT ( 'NONE',  ( 19.84048017005180142, -4.485898010009481851, -15.33043091644288225 ) ) ;
#19852=EDGE_LOOP ( 'NONE', ( #18559, #4961, #4735, #16271, #12060, #1439, #17543 ) ) ;
#19902=CARTESIAN_POINT ( 'NONE',  ( 19.80365268258534783, -6.408106014325641198, -14.04632085989190493 ) ) ;
#19908=ADVANCED_FACE ( 'NONE', ( #18184 ), #6456, .T. ) ;
#19930=CARTESIAN_POINT ( 'NONE',  ( 21.08189193827671915, -4.408480812526476278, -15.02976703352687693 ) ) ;
#19939=CARTESIAN_POINT ( 'NONE',  ( 11.68492118186053474, -0.1802169501065840895, -16.08014746593085320 ) ) ;
#19948=CARTESIAN_POINT ( 'NONE',  ( 12.36067866020131767, -0.4634977254221773757, -17.06924854999482832 ) ) ;
#19955=CARTESIAN_POINT ( 'NONE',  ( 18.58524860537636414, -6.287937115538260180, -15.54831227122795489 ) ) ;
#19969=ORIENTED_EDGE ( 'NONE', *, *, #13554, .T. ) ;
#20014=CARTESIAN_POINT ( 'NONE',  ( 8.776506035771831193, 2.891917824018316097, -16.46252061043899673 ) ) ;
#20034=CARTESIAN_POINT ( 'NONE',  ( 19.43502434582083183, -5.355863433658462291, -14.20139972047578958 ) ) ;
#20044=CARTESIAN_POINT ( 'NONE',  ( 14.45661145792178992, 1.227394729573359822, -16.40995970328339126 ) ) ;
#20052=CARTESIAN_POINT ( 'NONE',  ( 11.87648273465751281, -3.010377447276169072, -16.82793462644801963 ) ) ;
#20082=DIRECTION ( 'NONE',  ( -0.3697464814795229371, 0.9291326812858928808, 0.000000000000000000 ) ) ;
#20129=CARTESIAN_POINT ( 'NONE',  ( 11.57088620211501784, -5.974813487921917243, -17.02130989707151443 ) ) ;
#20141=CARTESIAN_POINT ( 'NONE',  ( 12.36142327289271847, -0.5412543480279620178, -16.62211206573401512 ) ) ;
#20158=CARTESIAN_POINT ( 'NONE',  ( 11.92901707314742410, -2.323620650010280286, -16.78204014074711381 ) ) ;
#20199=CARTESIAN_POINT ( 'NONE',  ( 17.33954469767427042, -6.884990403521952906, -14.58504387362480337 ) ) ;
#20210=VECTOR ( 'NONE', #12635, 1000.000000000000000 ) ;
#20215=EDGE_CURVE ( 'NONE', #20548, #9259, #18436, .T. ) ;
#20238=CARTESIAN_POINT ( 'NONE',  ( 19.75589755847548190, 0.01053015255646662547, -14.87810992461211335 ) ) ;
#20242=CARTESIAN_POINT ( 'NONE',  ( 10.72896046581951701, -3.334328103274969202, -17.13545616160453733 ) ) ;
#20247=CYLINDRICAL_SURFACE ( 'NONE', #21584, 0.5953125000000000222 ) ;
#20265=CARTESIAN_POINT ( 'NONE',  ( 12.23456664944783512, -4.754397903027896000, -16.81998147949391509 ) ) ;
#20298=CARTESIAN_POINT ( 'NONE',  ( 18.01622421214525360, -6.506453053838762379, -14.44805177597193691 ) ) ;
#20303=CYLINDRICAL_SURFACE ( 'NONE', #18773, 0.5953125000000000222 ) ;
#20342=CARTESIAN_POINT ( 'NONE',  ( 19.69476243405869198, 0.1068750216841468093, -14.89306782011991181 ) ) ;
#20346=CARTESIAN_POINT ( 'NONE',  ( 11.73031006892683692, -6.200208593250644995, -16.99046436023803963 ) ) ;
#20353=CARTESIAN_POINT ( 'NONE',  ( 20.07032048071632957, -2.740790541356518339, -14.17576409110674795 ) ) ;
#20371=CARTESIAN_POINT ( 'NONE',  ( 15.88496000606677150, -7.236326715571298251, -16.10278160673554382 ) ) ;
#20401=CARTESIAN_POINT ( 'NONE',  ( 14.92182958034182860, -7.164932238483936011, -15.08823842692338246 ) ) ;
#20452=CARTESIAN_POINT ( 'NONE',  ( 10.81663693033208062, -4.065912185102875220, -17.13981703108838062 ) ) ;
#20460=CARTESIAN_POINT ( 'NONE',  ( 20.23508918937977796, -1.359453322992689506, -14.75410208910826704 ) ) ;
#20464=CARTESIAN_POINT ( 'NONE',  ( 17.45896113601822464, -7.135217023119321489, -14.60636223679974499 ) ) ;
#20474=CARTESIAN_POINT ( 'NONE',  ( 14.12745558458436435, 2.161156110892227034, -16.49458891264261950 ) ) ;
#20482=CARTESIAN_POINT ( 'NONE',  ( 18.56537198735102123, -0.02379517359284155642, -14.65636392506457319 ) ) ;
#20483=PRODUCT_DEFINITION_CONTEXT ( 'detailed design', #17231, 'design' ) ;
#20518=CARTESIAN_POINT ( 'NONE',  ( 17.50089948725670652, -6.812435342835657437, -14.55200422611872391 ) ) ;
#20546=CARTESIAN_POINT ( 'NONE',  ( 20.95867805244277093, -1.145892873419149582, -15.34329086427974431 ) ) ;
#20548=VERTEX_POINT ( 'NONE', #13106 ) ;
#20572=CARTESIAN_POINT ( 'NONE',  ( 20.14958246138351683, -0.8772606718903691592, -14.78307071614850443 ) ) ;
#20593=CARTESIAN_POINT ( 'NONE',  ( 10.72591792739401306, -3.807102432456875629, -16.40592623193944632 ) ) ;
#20601=CARTESIAN_POINT ( 'NONE',  ( 14.36425966490409500, 0.8012915925827215347, -15.95786335565876968 ) ) ;
#20617=EDGE_CURVE ( 'NONE', #288, #11296, #13261, .T. ) ;
#20632=CARTESIAN_POINT ( 'NONE',  ( 18.57850393197893624, -6.030482575976392035, -14.33843453756632158 ) ) ;
#20640=CARTESIAN_POINT ( 'NONE',  ( 10.44501673953377896, -3.826156291150850652, -15.85328698979687445 ) ) ;
#20642=VERTEX_POINT ( 'NONE', #3009 ) ;
#20654=ORIENTED_EDGE ( 'NONE', *, *, #797, .F. ) ;
#20687=CARTESIAN_POINT ( 'NONE',  ( 20.16553087357842244, -0.1900022357140263018, -14.19585043658483237 ) ) ;
#20704=CARTESIAN_POINT ( 'NONE',  ( 13.99792333881812212, 2.297051954170742150, -16.18942158505737794 ) ) ;
#20712=LINE ( 'NONE', #5138, #5281 ) ;
#20732=CARTESIAN_POINT ( 'NONE',  ( 14.60682252872488540, -7.260664136960075510, -16.51448333835476490 ) ) ;
#20742=CARTESIAN_POINT ( 'NONE',  ( 21.58673283863862125, -3.402115365398042268, -14.98991958019304072 ) ) ;
#20744=DIRECTION ( 'NONE',  ( 0.2490110332224869660, 9.093548366658288884E-16, -0.9685006480810788299 ) ) ;
#20755=CARTESIAN_POINT ( 'NONE',  ( 21.01748975371211259, -1.169157164984415465, -15.02132963540784694 ) ) ;
#20795=CARTESIAN_POINT ( 'NONE',  ( 17.76390347290949379, 1.904479906339193507, -14.93461845486462458 ) ) ;
#20806=PRODUCT_CONTEXT ( 'NONE', #9318, 'mechanical' ) ;
#20809=MANIFOLD_SOLID_BREP ( 'Stock-MAS-676-1', #40 ) ;
#20810=CARTESIAN_POINT ( 'NONE',  ( 14.16117470977285109, -8.465632521890594120, -16.45114775117519912 ) ) ;
#20818=CARTESIAN_POINT ( 'NONE',  ( 19.71042948723761867, -2.147631015047439362, -14.24545724219409770 ) ) ;
#20822=ORIENTED_EDGE ( 'NONE', *, *, #10471, .F. ) ;
#20823=EDGE_CURVE ( 'NONE', #624, #288, #13796, .T. ) ;
#20839=CARTESIAN_POINT ( 'NONE',  ( 17.23303716620361214, -7.327103372956576877, -15.95966167909989508 ) ) ;
#20849=CARTESIAN_POINT ( 'NONE',  ( 20.23508736156870569, -1.359449706705495364, -14.75410053729980397 ) ) ;
#20851=CARTESIAN_POINT ( 'NONE',  ( 17.55504807725674965, -8.549671308339609865, -15.78569734679938996 ) ) ;
#20917=CARTESIAN_POINT ( 'NONE',  ( 11.56302892044394248, -0.1067246172791157244, -16.79663542313268465 ) ) ;
#20944=DIRECTION ( 'NONE',  ( -0.2490110332224855227, 0.000000000000000000, 0.9685006480810791629 ) ) ;
#20947=CARTESIAN_POINT ( 'NONE',  ( 14.81518831363163358, 0.9547697385890643318, -15.81862495919960487 ) ) ;
#20948=UNCERTAINTY_MEASURE_WITH_UNIT (LENGTH_MEASURE( 1.000000000000000082E-05 ), #3435, 'distance_accuracy_value', 'NONE');
#20963=CARTESIAN_POINT ( 'NONE',  ( 19.37805486502776375, 0.2182193654363457358, -15.04364546347907172 ) ) ;
#20966=CARTESIAN_POINT ( 'NONE',  ( 17.35374163439162132, -7.465977657333252360, -16.26709871504590410 ) ) ;
#20970=CARTESIAN_POINT ( 'NONE',  ( 20.92131311655350245, -1.145359114192535888, -15.19233952661473097 ) ) ;
#21007=FACE_OUTER_BOUND ( 'NONE', #7058, .T. ) ;
#21029=CARTESIAN_POINT ( 'NONE',  ( 11.72699871342261169, 0.1411900731644356866, -16.74345117411255401 ) ) ;
#21061=SHAPE_REPRESENTATION_RELATIONSHIP ( 'NONE' , 'NONE' ,  #11147, #1381 ) ;
#21066=CARTESIAN_POINT ( 'NONE',  ( 12.33924171467970154, -0.5403633132482419388, -16.54107158940488986 ) ) ;
#21079=CARTESIAN_POINT ( 'NONE',  ( 17.92763173077782923, -8.291096309418946930, -14.38181802688392175 ) ) ;
#21084=ORIENTED_EDGE ( 'NONE', *, *, #573, .F. ) ;
#21100=EDGE_LOOP ( 'NONE', ( #1749, #4071, #7360, #15831, #5079 ) ) ;
#21105=CARTESIAN_POINT ( 'NONE',  ( 13.52848780941367934, 19.04150370632758182, -20.24560135404512451 ) ) ;
#21127=CARTESIAN_POINT ( 'NONE',  ( 11.62205894965410913, -0.01747396230990239108, -16.77748880035451151 ) ) ;
#21143=ORIENTED_EDGE ( 'NONE', *, *, #20215, .F. ) ;
#21156=CARTESIAN_POINT ( 'NONE',  ( 11.64611064670678964, -6.985072876733208425, -15.86009521399990518 ) ) ;
#21162=CARTESIAN_POINT ( 'NONE',  ( 17.38991127515316393, -8.420206286881226632, -15.29446703135092633 ) ) ;
#21169=AXIS2_PLACEMENT_3D ( 'NONE', #21715, #13330, #4703 ) ;
#21172=CARTESIAN_POINT ( 'NONE',  ( 20.34285548276758604, -3.328947532601270964, -15.22298867112224485 ) ) ;
#21239=CARTESIAN_POINT ( 'NONE',  ( 13.94526350254431080, -8.131198800652363445, -15.30999825101322820 ) ) ;
#21266=CARTESIAN_POINT ( 'NONE',  ( 21.23967064989561493, -3.382426365437452009, -15.02713005365007959 ) ) ;
#21276=CARTESIAN_POINT ( 'NONE',  ( 20.45077234916881892, -6.011631478081029378, -13.76232490753369397 ) ) ;
#21345=CARTESIAN_POINT ( 'NONE',  ( 11.39261545403312326, -6.154307413984438035, -15.84502314252291733 ) ) ;
#21372=CARTESIAN_POINT ( 'NONE',  ( 20.51158336189590869, -5.799430522514935404, -15.12126906808022575 ) ) ;
#21383=EDGE_CURVE ( 'NONE', #14268, #8439, #6449, .T. ) ;
#21384=CARTESIAN_POINT ( 'NONE',  ( 11.59212630941054023, -6.991794502677832313, -15.67875784842310338 ) ) ;
#21390=CARTESIAN_POINT ( 'NONE',  ( 19.45582853530259371, 0.02454099089219423033, -15.02042049756312281 ) ) ;
#21392=CARTESIAN_POINT ( 'NONE',  ( 17.28264852343957969, 1.821796179831712603, -15.76246644883694614 ) ) ;
#21398=CARTESIAN_POINT ( 'NONE',  ( 19.42743112357013757, -5.337970718820712612, -15.39200997442386409 ) ) ;
#21405=CARTESIAN_POINT ( 'NONE',  ( 14.57357923071240791, -8.662971838486674514, -15.12377395242994282 ) ) ;
#21416=DIRECTION ( 'NONE',  ( -0.3482992169606098365, 0.9330960544336215357, -0.08955115110948595747 ) ) ;
#21451=CARTESIAN_POINT ( 'NONE',  ( 14.22686132395239156, -8.224742894641035917, -15.24862271894013865 ) ) ;
#21453=ORIENTED_EDGE ( 'NONE', *, *, #6648, .T. ) ;
#21476=CARTESIAN_POINT ( 'NONE',  ( 20.11748764637184905, -6.374101614863125320, -15.19701450337229076 ) ) ;
#21487=CARTESIAN_POINT ( 'NONE',  ( 14.01160604672443100, 1.694280624689696868, -15.36152992422168317 ) ) ;
#21497=CARTESIAN_POINT ( 'NONE',  ( 12.24295241119947519, -6.551777560806527845, -16.33579826273126301 ) ) ;
#21505=CARTESIAN_POINT ( 'NONE',  ( 19.10695511661582202, -5.767362265322653947, -15.44912671492631517 ) ) ;
#21565=CARTESIAN_POINT ( 'NONE',  ( 20.55406668138206427, -5.109279823642991936, -13.90851210264134075 ) ) ;
#21584=AXIS2_PLACEMENT_3D ( 'NONE', #8982, #7332, #10429 ) ;
#21603=CARTESIAN_POINT ( 'NONE',  ( 12.22927362527537731, -5.743469473357618149, -16.38050967881292053 ) ) ;
#21621=CARTESIAN_POINT ( 'NONE',  ( 14.46430160870318460, -6.938395347649755962, -16.39814615911750550 ) ) ;
#21678=DIRECTION ( 'NONE',  ( -0.3697464814795228816, 0.9291326812858931028, 0.000000000000000000 ) ) ;
#21705=CARTESIAN_POINT ( 'NONE',  ( 21.21167325040990903, -2.309581742399265281, -15.07358112151901963 ) ) ;
#21715=CARTESIAN_POINT ( 'NONE',  ( 14.14084833952063747, 15.36419388438619649, -16.93566361603518899 ) ) ;
#21717=CARTESIAN_POINT ( 'NONE',  ( 14.54316325888261119, -8.043841742527851224, -14.50243733777968380 ) ) ;
#21726=CARTESIAN_POINT ( 'NONE',  ( 11.62054768543827166, -3.675972292006682185, -16.17590813040945008 ) ) ;
#21731=AXIS2_PLACEMENT_3D ( 'NONE', #13418, #5004, #16423 ) ;
#21732=CARTESIAN_POINT ( 'NONE',  ( 14.82108974844347848, -7.069631093989277915, -16.32458675325787922 ) ) ;
#21773=CARTESIAN_POINT ( 'NONE',  ( 13.62051399351888747, 17.23237496650334677, -17.80340391586448234 ) ) ;
#21805=CARTESIAN_POINT ( 'NONE',  ( 15.81640869719298870, -8.433271052806768253, -16.11895057086533356 ) ) ;
#21815=DIRECTION ( 'NONE',  ( -0.3482992169606098365, 0.9330960544336215357, -0.08955115110948595747 ) ) ;
#21816=CARTESIAN_POINT ( 'NONE',  ( 12.42461531891860105, -5.659038248882215072, -16.66875675070026830 ) ) ;
#21828=CARTESIAN_POINT ( 'NONE',  ( 14.20148524362829257, -8.473402551277725792, -16.61869953724475124 ) ) ;
#21834=CARTESIAN_POINT ( 'NONE',  ( 12.06866590677377005, -4.286523879175909713, -16.83933591760442283 ) ) ;
#21857=DIRECTION ( 'NONE',  ( -0.9037041334408600912, -0.3596272420165190775, -0.2323512126103423614 ) ) ;
ENDSEC;
END-ISO-10303-21;
